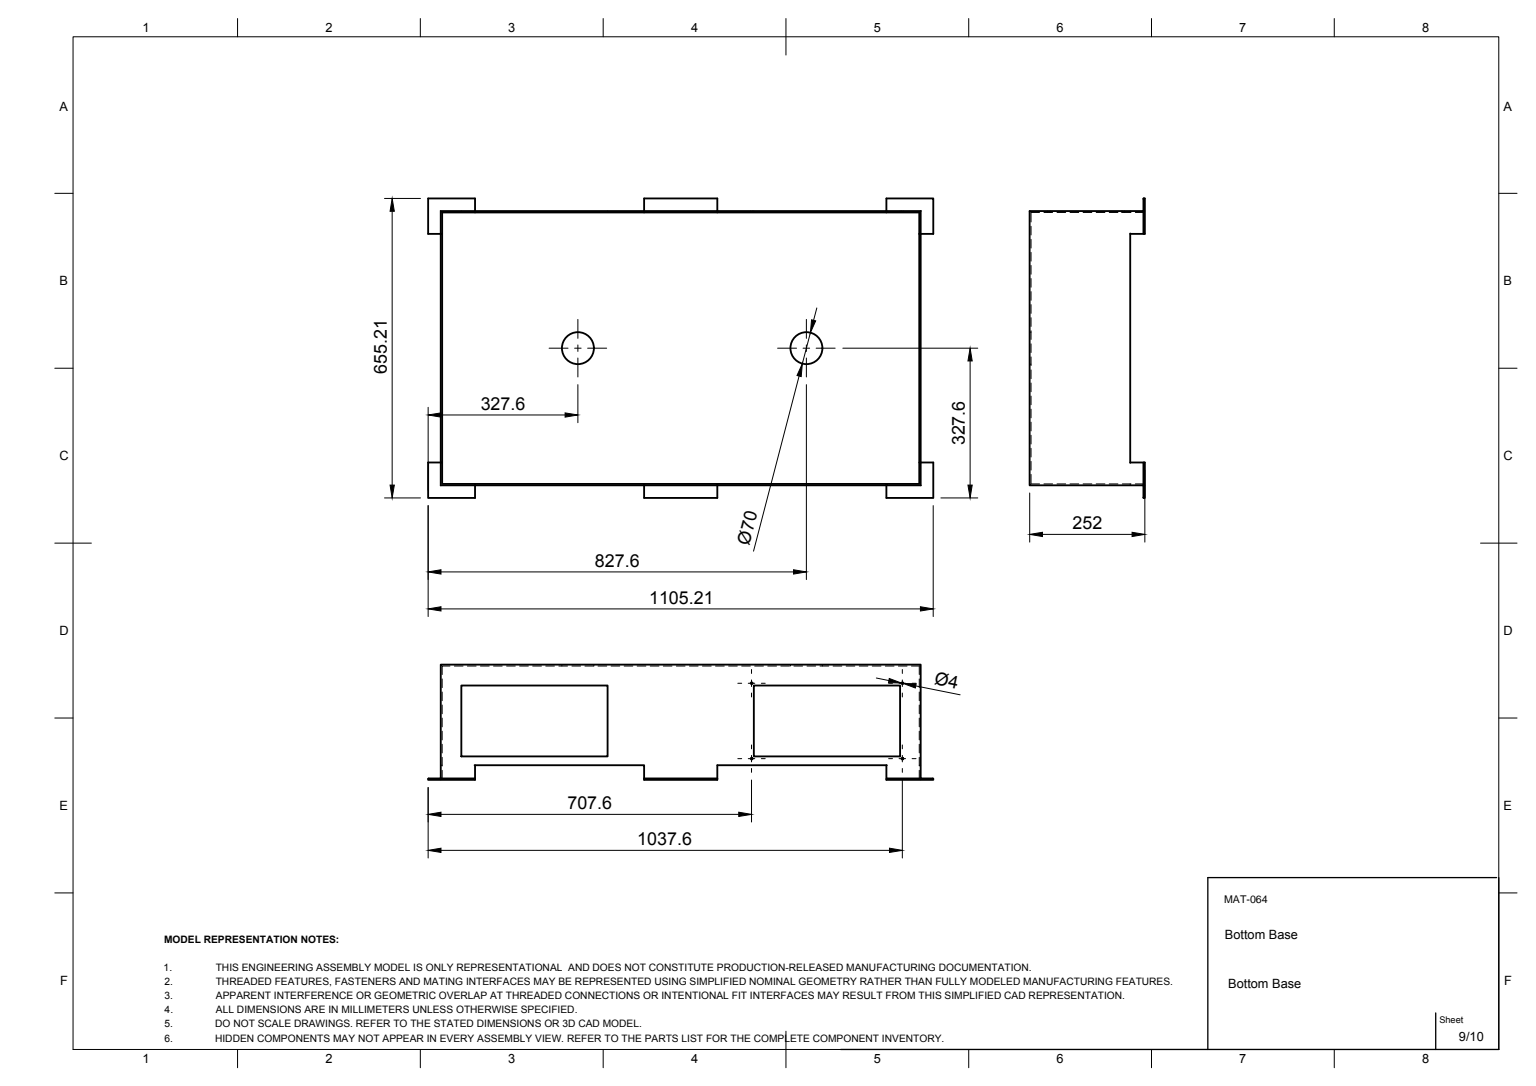
ISO-10303-21;
HEADER;
/* Generated by software containing ST-Developer
 * from STEP Tools, Inc. (www.steptools.com) 
 */

FILE_DESCRIPTION(
/* description */ (''),
/* implementation_level */ '2;1');

FILE_NAME(
/* name */ 
'Bottom Base.step',
/* time_stamp */ '2026-10-24T12:42:14-07:00',
/* author */ (''),
/* organization */ (''),
/* preprocessor_version */ 'ST-DEVELOPER v20.2',
/* originating_system */ 'Autodesk Translation Framework v15.15.0.0',
/* authorisation */ '');

FILE_SCHEMA (('AUTOMOTIVE_DESIGN { 1 0 10303 214 3 1 1 }'));
ENDSEC;

DATA;
#10=MECHANICAL_DESIGN_GEOMETRIC_PRESENTATION_REPRESENTATION('',(#66),#6789);
#54=SHAPE_REPRESENTATION_RELATIONSHIP('SRR','None',#6821,#60);
#60=ADVANCED_BREP_SHAPE_REPRESENTATION('',(#72),#6783);
#66=STYLED_ITEM('',(#6863),#72);
#72=MANIFOLD_SOLID_BREP('Bottom Base',#3961);
#78=TOROIDAL_SURFACE('',#4150,2.,1.);
#79=TOROIDAL_SURFACE('',#4160,2.,1.);
#80=TOROIDAL_SURFACE('',#4170,2.,1.);
#81=TOROIDAL_SURFACE('',#4180,2.,1.);
#82=TOROIDAL_SURFACE('',#4190,2.,1.);
#83=TOROIDAL_SURFACE('',#4200,2.,1.);
#84=TOROIDAL_SURFACE('',#4208,2.,1.);
#85=TOROIDAL_SURFACE('',#4220,2.,1.);
#92=ELLIPSE('',#4145,1.41421356237309,1.);
#93=ELLIPSE('',#4149,1.41421356237309,1.);
#94=ELLIPSE('',#4153,1.41421356237309,1.);
#95=ELLIPSE('',#4155,1.41421356237309,1.);
#96=ELLIPSE('',#4165,1.4142135623731,1.);
#97=ELLIPSE('',#4169,1.41421356237309,1.);
#98=ELLIPSE('',#4173,1.41421356237309,1.);
#99=ELLIPSE('',#4175,1.41421356237309,1.);
#100=ELLIPSE('',#4185,1.41421356237309,1.);
#101=ELLIPSE('',#4189,1.41421356237309,1.);
#102=ELLIPSE('',#4193,1.41421356237309,1.);
#103=ELLIPSE('',#4195,1.41421356237309,1.);
#104=ELLIPSE('',#4206,1.41421356237309,1.);
#105=ELLIPSE('',#4211,1.41421356237309,1.);
#106=ELLIPSE('',#4213,1.4142135623731,1.);
#107=ELLIPSE('',#4215,1.4142135623731,1.);
#108=CYLINDRICAL_SURFACE('',#4093,2.);
#109=CYLINDRICAL_SURFACE('',#4094,2.);
#110=CYLINDRICAL_SURFACE('',#4095,2.);
#111=CYLINDRICAL_SURFACE('',#4096,2.);
#112=CYLINDRICAL_SURFACE('',#4143,1.);
#113=CYLINDRICAL_SURFACE('',#4146,1.);
#114=CYLINDRICAL_SURFACE('',#4148,1.);
#115=CYLINDRICAL_SURFACE('',#4152,1.);
#116=CYLINDRICAL_SURFACE('',#4154,1.);
#117=CYLINDRICAL_SURFACE('',#4156,1.);
#118=CYLINDRICAL_SURFACE('',#4158,1.);
#119=CYLINDRICAL_SURFACE('',#4162,1.);
#120=CYLINDRICAL_SURFACE('',#4163,1.);
#121=CYLINDRICAL_SURFACE('',#4166,1.);
#122=CYLINDRICAL_SURFACE('',#4168,1.);
#123=CYLINDRICAL_SURFACE('',#4172,1.);
#124=CYLINDRICAL_SURFACE('',#4174,1.);
#125=CYLINDRICAL_SURFACE('',#4176,1.);
#126=CYLINDRICAL_SURFACE('',#4178,1.);
#127=CYLINDRICAL_SURFACE('',#4182,1.);
#128=CYLINDRICAL_SURFACE('',#4183,1.);
#129=CYLINDRICAL_SURFACE('',#4186,1.);
#130=CYLINDRICAL_SURFACE('',#4188,1.);
#131=CYLINDRICAL_SURFACE('',#4192,1.);
#132=CYLINDRICAL_SURFACE('',#4194,1.);
#133=CYLINDRICAL_SURFACE('',#4196,1.);
#134=CYLINDRICAL_SURFACE('',#4198,1.);
#135=CYLINDRICAL_SURFACE('',#4202,1.);
#136=CYLINDRICAL_SURFACE('',#4203,1.);
#137=CYLINDRICAL_SURFACE('',#4205,1.);
#138=CYLINDRICAL_SURFACE('',#4210,1.);
#139=CYLINDRICAL_SURFACE('',#4212,1.);
#140=CYLINDRICAL_SURFACE('',#4214,1.);
#141=CYLINDRICAL_SURFACE('',#4216,1.);
#142=CYLINDRICAL_SURFACE('',#4218,1.);
#143=CYLINDRICAL_SURFACE('',#4222,1.);
#144=CYLINDRICAL_SURFACE('',#4223,35.);
#145=CYLINDRICAL_SURFACE('',#4224,35.);
#185=FACE_BOUND('',#612,.T.);
#186=FACE_BOUND('',#613,.T.);
#187=FACE_BOUND('',#614,.T.);
#188=FACE_BOUND('',#615,.T.);
#189=FACE_BOUND('',#616,.T.);
#190=FACE_BOUND('',#617,.T.);
#191=FACE_BOUND('',#624,.T.);
#192=FACE_BOUND('',#625,.T.);
#193=FACE_BOUND('',#626,.T.);
#194=FACE_BOUND('',#627,.T.);
#195=FACE_BOUND('',#628,.T.);
#196=FACE_BOUND('',#629,.T.);
#197=FACE_BOUND('',#635,.T.);
#198=FACE_BOUND('',#636,.T.);
#199=FACE_BOUND('',#641,.T.);
#200=FACE_BOUND('',#642,.T.);
#242=CIRCLE('',#4038,2.);
#243=CIRCLE('',#4039,2.);
#244=CIRCLE('',#4040,2.);
#245=CIRCLE('',#4041,2.);
#246=CIRCLE('',#4048,2.);
#247=CIRCLE('',#4049,2.);
#248=CIRCLE('',#4050,2.);
#249=CIRCLE('',#4051,2.);
#250=CIRCLE('',#4057,35.);
#251=CIRCLE('',#4058,35.);
#252=CIRCLE('',#4063,35.);
#253=CIRCLE('',#4064,35.);
#254=CIRCLE('',#4067,1.);
#255=CIRCLE('',#4069,2.);
#256=CIRCLE('',#4071,2.);
#257=CIRCLE('',#4073,1.);
#258=CIRCLE('',#4077,1.);
#259=CIRCLE('',#4079,2.);
#260=CIRCLE('',#4082,2.);
#261=CIRCLE('',#4084,1.);
#262=CIRCLE('',#4098,2.);
#263=CIRCLE('',#4100,1.);
#264=CIRCLE('',#4101,1.);
#265=CIRCLE('',#4103,2.);
#266=CIRCLE('',#4105,2.);
#267=CIRCLE('',#4107,1.);
#268=CIRCLE('',#4108,1.);
#269=CIRCLE('',#4110,2.);
#270=CIRCLE('',#4144,1.);
#271=CIRCLE('',#4147,1.);
#272=CIRCLE('',#4151,1.);
#273=CIRCLE('',#4157,1.);
#274=CIRCLE('',#4159,1.);
#275=CIRCLE('',#4161,1.);
#276=CIRCLE('',#4164,1.);
#277=CIRCLE('',#4167,1.);
#278=CIRCLE('',#4171,1.);
#279=CIRCLE('',#4177,1.);
#280=CIRCLE('',#4179,1.);
#281=CIRCLE('',#4181,1.);
#282=CIRCLE('',#4184,1.);
#283=CIRCLE('',#4187,1.);
#284=CIRCLE('',#4191,1.);
#285=CIRCLE('',#4197,1.);
#286=CIRCLE('',#4199,1.);
#287=CIRCLE('',#4201,1.);
#288=CIRCLE('',#4204,1.);
#289=CIRCLE('',#4207,1.);
#290=CIRCLE('',#4209,1.);
#291=CIRCLE('',#4217,1.);
#292=CIRCLE('',#4219,1.);
#293=CIRCLE('',#4221,1.);
#394=FACE_OUTER_BOUND('',#611,.T.);
#395=FACE_OUTER_BOUND('',#618,.T.);
#396=FACE_OUTER_BOUND('',#619,.T.);
#397=FACE_OUTER_BOUND('',#620,.T.);
#398=FACE_OUTER_BOUND('',#621,.T.);
#399=FACE_OUTER_BOUND('',#622,.T.);
#400=FACE_OUTER_BOUND('',#623,.T.);
#401=FACE_OUTER_BOUND('',#630,.T.);
#402=FACE_OUTER_BOUND('',#631,.T.);
#403=FACE_OUTER_BOUND('',#632,.T.);
#404=FACE_OUTER_BOUND('',#633,.T.);
#405=FACE_OUTER_BOUND('',#634,.T.);
#406=FACE_OUTER_BOUND('',#637,.T.);
#407=FACE_OUTER_BOUND('',#638,.T.);
#408=FACE_OUTER_BOUND('',#639,.T.);
#409=FACE_OUTER_BOUND('',#640,.T.);
#410=FACE_OUTER_BOUND('',#643,.T.);
#411=FACE_OUTER_BOUND('',#644,.T.);
#412=FACE_OUTER_BOUND('',#645,.T.);
#413=FACE_OUTER_BOUND('',#646,.T.);
#414=FACE_OUTER_BOUND('',#647,.T.);
#415=FACE_OUTER_BOUND('',#648,.T.);
#416=FACE_OUTER_BOUND('',#649,.T.);
#417=FACE_OUTER_BOUND('',#650,.T.);
#418=FACE_OUTER_BOUND('',#651,.T.);
#419=FACE_OUTER_BOUND('',#652,.T.);
#420=FACE_OUTER_BOUND('',#653,.T.);
#421=FACE_OUTER_BOUND('',#654,.T.);
#422=FACE_OUTER_BOUND('',#655,.T.);
#423=FACE_OUTER_BOUND('',#656,.T.);
#424=FACE_OUTER_BOUND('',#657,.T.);
#425=FACE_OUTER_BOUND('',#658,.T.);
#426=FACE_OUTER_BOUND('',#659,.T.);
#427=FACE_OUTER_BOUND('',#660,.T.);
#428=FACE_OUTER_BOUND('',#661,.T.);
#429=FACE_OUTER_BOUND('',#662,.T.);
#430=FACE_OUTER_BOUND('',#663,.T.);
#431=FACE_OUTER_BOUND('',#664,.T.);
#432=FACE_OUTER_BOUND('',#665,.T.);
#433=FACE_OUTER_BOUND('',#666,.T.);
#434=FACE_OUTER_BOUND('',#667,.T.);
#435=FACE_OUTER_BOUND('',#668,.T.);
#436=FACE_OUTER_BOUND('',#669,.T.);
#437=FACE_OUTER_BOUND('',#670,.T.);
#438=FACE_OUTER_BOUND('',#671,.T.);
#439=FACE_OUTER_BOUND('',#672,.T.);
#440=FACE_OUTER_BOUND('',#673,.T.);
#441=FACE_OUTER_BOUND('',#674,.T.);
#442=FACE_OUTER_BOUND('',#675,.T.);
#443=FACE_OUTER_BOUND('',#676,.T.);
#444=FACE_OUTER_BOUND('',#677,.T.);
#445=FACE_OUTER_BOUND('',#678,.T.);
#446=FACE_OUTER_BOUND('',#679,.T.);
#447=FACE_OUTER_BOUND('',#680,.T.);
#448=FACE_OUTER_BOUND('',#681,.T.);
#449=FACE_OUTER_BOUND('',#682,.T.);
#450=FACE_OUTER_BOUND('',#683,.T.);
#451=FACE_OUTER_BOUND('',#684,.T.);
#452=FACE_OUTER_BOUND('',#685,.T.);
#453=FACE_OUTER_BOUND('',#686,.T.);
#454=FACE_OUTER_BOUND('',#687,.T.);
#455=FACE_OUTER_BOUND('',#688,.T.);
#456=FACE_OUTER_BOUND('',#689,.T.);
#457=FACE_OUTER_BOUND('',#690,.T.);
#458=FACE_OUTER_BOUND('',#691,.T.);
#459=FACE_OUTER_BOUND('',#692,.T.);
#460=FACE_OUTER_BOUND('',#693,.T.);
#461=FACE_OUTER_BOUND('',#694,.T.);
#462=FACE_OUTER_BOUND('',#695,.T.);
#463=FACE_OUTER_BOUND('',#696,.T.);
#464=FACE_OUTER_BOUND('',#697,.T.);
#465=FACE_OUTER_BOUND('',#698,.T.);
#466=FACE_OUTER_BOUND('',#699,.T.);
#467=FACE_OUTER_BOUND('',#700,.T.);
#468=FACE_OUTER_BOUND('',#701,.T.);
#469=FACE_OUTER_BOUND('',#702,.T.);
#470=FACE_OUTER_BOUND('',#703,.T.);
#471=FACE_OUTER_BOUND('',#704,.T.);
#472=FACE_OUTER_BOUND('',#705,.T.);
#473=FACE_OUTER_BOUND('',#706,.T.);
#474=FACE_OUTER_BOUND('',#707,.T.);
#475=FACE_OUTER_BOUND('',#708,.T.);
#476=FACE_OUTER_BOUND('',#709,.T.);
#477=FACE_OUTER_BOUND('',#710,.T.);
#478=FACE_OUTER_BOUND('',#711,.T.);
#479=FACE_OUTER_BOUND('',#712,.T.);
#480=FACE_OUTER_BOUND('',#713,.T.);
#481=FACE_OUTER_BOUND('',#714,.T.);
#482=FACE_OUTER_BOUND('',#715,.T.);
#483=FACE_OUTER_BOUND('',#716,.T.);
#484=FACE_OUTER_BOUND('',#717,.T.);
#485=FACE_OUTER_BOUND('',#718,.T.);
#486=FACE_OUTER_BOUND('',#719,.T.);
#487=FACE_OUTER_BOUND('',#720,.T.);
#488=FACE_OUTER_BOUND('',#721,.T.);
#489=FACE_OUTER_BOUND('',#722,.T.);
#490=FACE_OUTER_BOUND('',#723,.T.);
#491=FACE_OUTER_BOUND('',#724,.T.);
#492=FACE_OUTER_BOUND('',#725,.T.);
#493=FACE_OUTER_BOUND('',#726,.T.);
#494=FACE_OUTER_BOUND('',#727,.T.);
#495=FACE_OUTER_BOUND('',#728,.T.);
#496=FACE_OUTER_BOUND('',#729,.T.);
#497=FACE_OUTER_BOUND('',#730,.T.);
#498=FACE_OUTER_BOUND('',#731,.T.);
#499=FACE_OUTER_BOUND('',#732,.T.);
#500=FACE_OUTER_BOUND('',#733,.T.);
#501=FACE_OUTER_BOUND('',#734,.T.);
#502=FACE_OUTER_BOUND('',#735,.T.);
#503=FACE_OUTER_BOUND('',#736,.T.);
#504=FACE_OUTER_BOUND('',#737,.T.);
#505=FACE_OUTER_BOUND('',#738,.T.);
#506=FACE_OUTER_BOUND('',#739,.T.);
#507=FACE_OUTER_BOUND('',#740,.T.);
#508=FACE_OUTER_BOUND('',#741,.T.);
#509=FACE_OUTER_BOUND('',#742,.T.);
#510=FACE_OUTER_BOUND('',#743,.T.);
#511=FACE_OUTER_BOUND('',#744,.T.);
#512=FACE_OUTER_BOUND('',#745,.T.);
#513=FACE_OUTER_BOUND('',#746,.T.);
#611=EDGE_LOOP('',(#2533,#2534,#2535,#2536,#2537,#2538,#2539,#2540,#2541,
#2542,#2543,#2544));
#612=EDGE_LOOP('',(#2545));
#613=EDGE_LOOP('',(#2546));
#614=EDGE_LOOP('',(#2547));
#615=EDGE_LOOP('',(#2548));
#616=EDGE_LOOP('',(#2549,#2550,#2551,#2552));
#617=EDGE_LOOP('',(#2553,#2554,#2555,#2556));
#618=EDGE_LOOP('',(#2557,#2558,#2559,#2560,#2561,#2562,#2563,#2564));
#619=EDGE_LOOP('',(#2565,#2566,#2567,#2568,#2569,#2570,#2571,#2572,#2573,
#2574,#2575,#2576));
#620=EDGE_LOOP('',(#2577,#2578,#2579,#2580,#2581,#2582,#2583,#2584));
#621=EDGE_LOOP('',(#2585,#2586,#2587,#2588,#2589,#2590));
#622=EDGE_LOOP('',(#2591,#2592,#2593,#2594,#2595,#2596));
#623=EDGE_LOOP('',(#2597,#2598,#2599,#2600,#2601,#2602,#2603,#2604,#2605,
#2606,#2607,#2608));
#624=EDGE_LOOP('',(#2609,#2610,#2611,#2612));
#625=EDGE_LOOP('',(#2613));
#626=EDGE_LOOP('',(#2614));
#627=EDGE_LOOP('',(#2615));
#628=EDGE_LOOP('',(#2616));
#629=EDGE_LOOP('',(#2617,#2618,#2619,#2620));
#630=EDGE_LOOP('',(#2621,#2622,#2623,#2624));
#631=EDGE_LOOP('',(#2625,#2626,#2627,#2628));
#632=EDGE_LOOP('',(#2629,#2630,#2631,#2632,#2633,#2634));
#633=EDGE_LOOP('',(#2635,#2636,#2637,#2638,#2639,#2640));
#634=EDGE_LOOP('',(#2641,#2642,#2643,#2644));
#635=EDGE_LOOP('',(#2645));
#636=EDGE_LOOP('',(#2646));
#637=EDGE_LOOP('',(#2647,#2648,#2649,#2650,#2651,#2652,#2653,#2654));
#638=EDGE_LOOP('',(#2655,#2656,#2657,#2658,#2659,#2660,#2661,#2662,#2663,
#2664,#2665,#2666));
#639=EDGE_LOOP('',(#2667,#2668,#2669,#2670,#2671,#2672,#2673,#2674));
#640=EDGE_LOOP('',(#2675,#2676,#2677,#2678));
#641=EDGE_LOOP('',(#2679));
#642=EDGE_LOOP('',(#2680));
#643=EDGE_LOOP('',(#2681,#2682,#2683,#2684,#2685,#2686,#2687,#2688));
#644=EDGE_LOOP('',(#2689,#2690,#2691,#2692,#2693));
#645=EDGE_LOOP('',(#2694,#2695,#2696,#2697,#2698,#2699,#2700,#2701,#2702));
#646=EDGE_LOOP('',(#2703,#2704,#2705,#2706,#2707,#2708,#2709,#2710,#2711));
#647=EDGE_LOOP('',(#2712,#2713,#2714,#2715,#2716));
#648=EDGE_LOOP('',(#2717,#2718,#2719,#2720,#2721,#2722,#2723,#2724));
#649=EDGE_LOOP('',(#2725,#2726,#2727,#2728,#2729,#2730,#2731,#2732));
#650=EDGE_LOOP('',(#2733,#2734,#2735,#2736,#2737));
#651=EDGE_LOOP('',(#2738,#2739,#2740,#2741,#2742,#2743,#2744,#2745,#2746));
#652=EDGE_LOOP('',(#2747,#2748,#2749,#2750,#2751,#2752,#2753,#2754));
#653=EDGE_LOOP('',(#2755,#2756,#2757,#2758,#2759,#2760,#2761,#2762,#2763));
#654=EDGE_LOOP('',(#2764,#2765,#2766,#2767,#2768));
#655=EDGE_LOOP('',(#2769,#2770,#2771,#2772));
#656=EDGE_LOOP('',(#2773,#2774,#2775,#2776));
#657=EDGE_LOOP('',(#2777,#2778,#2779,#2780));
#658=EDGE_LOOP('',(#2781,#2782,#2783,#2784));
#659=EDGE_LOOP('',(#2785,#2786,#2787,#2788));
#660=EDGE_LOOP('',(#2789,#2790,#2791,#2792));
#661=EDGE_LOOP('',(#2793,#2794,#2795,#2796));
#662=EDGE_LOOP('',(#2797,#2798,#2799,#2800));
#663=EDGE_LOOP('',(#2801,#2802,#2803,#2804));
#664=EDGE_LOOP('',(#2805,#2806,#2807,#2808));
#665=EDGE_LOOP('',(#2809,#2810,#2811,#2812));
#666=EDGE_LOOP('',(#2813,#2814,#2815,#2816));
#667=EDGE_LOOP('',(#2817,#2818,#2819,#2820,#2821,#2822,#2823,#2824,#2825));
#668=EDGE_LOOP('',(#2826,#2827,#2828,#2829,#2830,#2831));
#669=EDGE_LOOP('',(#2832,#2833,#2834,#2835,#2836,#2837,#2838,#2839,#2840));
#670=EDGE_LOOP('',(#2841,#2842,#2843,#2844,#2845,#2846,#2847,#2848,#2849));
#671=EDGE_LOOP('',(#2850,#2851,#2852,#2853,#2854,#2855));
#672=EDGE_LOOP('',(#2856,#2857,#2858,#2859,#2860,#2861,#2862,#2863,#2864));
#673=EDGE_LOOP('',(#2865,#2866,#2867,#2868));
#674=EDGE_LOOP('',(#2869,#2870,#2871,#2872));
#675=EDGE_LOOP('',(#2873,#2874,#2875,#2876));
#676=EDGE_LOOP('',(#2877,#2878,#2879,#2880));
#677=EDGE_LOOP('',(#2881,#2882,#2883,#2884,#2885,#2886));
#678=EDGE_LOOP('',(#2887,#2888,#2889,#2890,#2891,#2892));
#679=EDGE_LOOP('',(#2893,#2894,#2895,#2896));
#680=EDGE_LOOP('',(#2897,#2898,#2899,#2900));
#681=EDGE_LOOP('',(#2901,#2902,#2903,#2904));
#682=EDGE_LOOP('',(#2905,#2906,#2907,#2908));
#683=EDGE_LOOP('',(#2909,#2910,#2911,#2912,#2913,#2914));
#684=EDGE_LOOP('',(#2915,#2916,#2917,#2918,#2919,#2920));
#685=EDGE_LOOP('',(#2921,#2922,#2923,#2924));
#686=EDGE_LOOP('',(#2925,#2926,#2927,#2928));
#687=EDGE_LOOP('',(#2929,#2930,#2931,#2932));
#688=EDGE_LOOP('',(#2933,#2934,#2935,#2936));
#689=EDGE_LOOP('',(#2937,#2938,#2939,#2940,#2941,#2942));
#690=EDGE_LOOP('',(#2943,#2944,#2945,#2946,#2947,#2948));
#691=EDGE_LOOP('',(#2949,#2950,#2951,#2952));
#692=EDGE_LOOP('',(#2953,#2954,#2955,#2956));
#693=EDGE_LOOP('',(#2957,#2958,#2959,#2960));
#694=EDGE_LOOP('',(#2961,#2962,#2963,#2964));
#695=EDGE_LOOP('',(#2965,#2966,#2967,#2968,#2969,#2970));
#696=EDGE_LOOP('',(#2971,#2972,#2973,#2974,#2975,#2976));
#697=EDGE_LOOP('',(#2977,#2978,#2979,#2980));
#698=EDGE_LOOP('',(#2981,#2982,#2983,#2984));
#699=EDGE_LOOP('',(#2985,#2986,#2987,#2988));
#700=EDGE_LOOP('',(#2989,#2990,#2991,#2992));
#701=EDGE_LOOP('',(#2993,#2994,#2995,#2996));
#702=EDGE_LOOP('',(#2997,#2998,#2999,#3000));
#703=EDGE_LOOP('',(#3001,#3002,#3003,#3004));
#704=EDGE_LOOP('',(#3005,#3006,#3007,#3008));
#705=EDGE_LOOP('',(#3009,#3010,#3011,#3012));
#706=EDGE_LOOP('',(#3013,#3014,#3015,#3016));
#707=EDGE_LOOP('',(#3017,#3018,#3019,#3020));
#708=EDGE_LOOP('',(#3021,#3022,#3023,#3024));
#709=EDGE_LOOP('',(#3025,#3026,#3027,#3028));
#710=EDGE_LOOP('',(#3029,#3030,#3031,#3032));
#711=EDGE_LOOP('',(#3033,#3034,#3035,#3036));
#712=EDGE_LOOP('',(#3037,#3038,#3039,#3040));
#713=EDGE_LOOP('',(#3041,#3042,#3043,#3044));
#714=EDGE_LOOP('',(#3045,#3046,#3047,#3048));
#715=EDGE_LOOP('',(#3049,#3050,#3051,#3052));
#716=EDGE_LOOP('',(#3053,#3054,#3055,#3056));
#717=EDGE_LOOP('',(#3057,#3058,#3059,#3060));
#718=EDGE_LOOP('',(#3061,#3062,#3063,#3064));
#719=EDGE_LOOP('',(#3065,#3066,#3067,#3068));
#720=EDGE_LOOP('',(#3069,#3070,#3071,#3072));
#721=EDGE_LOOP('',(#3073,#3074,#3075,#3076));
#722=EDGE_LOOP('',(#3077,#3078,#3079,#3080));
#723=EDGE_LOOP('',(#3081,#3082,#3083,#3084));
#724=EDGE_LOOP('',(#3085,#3086,#3087,#3088));
#725=EDGE_LOOP('',(#3089,#3090,#3091,#3092));
#726=EDGE_LOOP('',(#3093,#3094,#3095,#3096));
#727=EDGE_LOOP('',(#3097,#3098,#3099,#3100));
#728=EDGE_LOOP('',(#3101,#3102,#3103,#3104));
#729=EDGE_LOOP('',(#3105,#3106,#3107,#3108));
#730=EDGE_LOOP('',(#3109,#3110,#3111,#3112));
#731=EDGE_LOOP('',(#3113,#3114,#3115,#3116));
#732=EDGE_LOOP('',(#3117,#3118,#3119,#3120));
#733=EDGE_LOOP('',(#3121,#3122,#3123,#3124));
#734=EDGE_LOOP('',(#3125,#3126,#3127,#3128));
#735=EDGE_LOOP('',(#3129,#3130,#3131,#3132));
#736=EDGE_LOOP('',(#3133,#3134,#3135,#3136));
#737=EDGE_LOOP('',(#3137,#3138,#3139,#3140));
#738=EDGE_LOOP('',(#3141,#3142,#3143,#3144));
#739=EDGE_LOOP('',(#3145,#3146,#3147,#3148));
#740=EDGE_LOOP('',(#3149,#3150,#3151,#3152));
#741=EDGE_LOOP('',(#3153,#3154,#3155,#3156));
#742=EDGE_LOOP('',(#3157,#3158,#3159,#3160));
#743=EDGE_LOOP('',(#3161,#3162,#3163,#3164));
#744=EDGE_LOOP('',(#3165,#3166,#3167,#3168));
#745=EDGE_LOOP('',(#3169,#3170,#3171,#3172));
#746=EDGE_LOOP('',(#3173,#3174,#3175,#3176));
#885=LINE('',#5612,#1263);
#886=LINE('',#5614,#1264);
#887=LINE('',#5616,#1265);
#888=LINE('',#5618,#1266);
#889=LINE('',#5620,#1267);
#890=LINE('',#5622,#1268);
#891=LINE('',#5624,#1269);
#892=LINE('',#5626,#1270);
#893=LINE('',#5628,#1271);
#894=LINE('',#5630,#1272);
#895=LINE('',#5632,#1273);
#896=LINE('',#5633,#1274);
#897=LINE('',#5644,#1275);
#898=LINE('',#5646,#1276);
#899=LINE('',#5648,#1277);
#900=LINE('',#5649,#1278);
#901=LINE('',#5652,#1279);
#902=LINE('',#5654,#1280);
#903=LINE('',#5656,#1281);
#904=LINE('',#5657,#1282);
#905=LINE('',#5661,#1283);
#906=LINE('',#5663,#1284);
#907=LINE('',#5665,#1285);
#908=LINE('',#5666,#1286);
#909=LINE('',#5668,#1287);
#910=LINE('',#5670,#1288);
#911=LINE('',#5671,#1289);
#912=LINE('',#5675,#1290);
#913=LINE('',#5677,#1291);
#914=LINE('',#5678,#1292);
#915=LINE('',#5680,#1293);
#916=LINE('',#5682,#1294);
#917=LINE('',#5684,#1295);
#918=LINE('',#5686,#1296);
#919=LINE('',#5688,#1297);
#920=LINE('',#5690,#1298);
#921=LINE('',#5692,#1299);
#922=LINE('',#5693,#1300);
#923=LINE('',#5697,#1301);
#924=LINE('',#5699,#1302);
#925=LINE('',#5700,#1303);
#926=LINE('',#5701,#1304);
#927=LINE('',#5703,#1305);
#928=LINE('',#5704,#1306);
#929=LINE('',#5708,#1307);
#930=LINE('',#5710,#1308);
#931=LINE('',#5712,#1309);
#932=LINE('',#5714,#1310);
#933=LINE('',#5716,#1311);
#934=LINE('',#5717,#1312);
#935=LINE('',#5721,#1313);
#936=LINE('',#5723,#1314);
#937=LINE('',#5725,#1315);
#938=LINE('',#5727,#1316);
#939=LINE('',#5729,#1317);
#940=LINE('',#5730,#1318);
#941=LINE('',#5734,#1319);
#942=LINE('',#5736,#1320);
#943=LINE('',#5738,#1321);
#944=LINE('',#5740,#1322);
#945=LINE('',#5742,#1323);
#946=LINE('',#5744,#1324);
#947=LINE('',#5746,#1325);
#948=LINE('',#5748,#1326);
#949=LINE('',#5750,#1327);
#950=LINE('',#5752,#1328);
#951=LINE('',#5754,#1329);
#952=LINE('',#5755,#1330);
#953=LINE('',#5758,#1331);
#954=LINE('',#5760,#1332);
#955=LINE('',#5762,#1333);
#956=LINE('',#5763,#1334);
#957=LINE('',#5774,#1335);
#958=LINE('',#5776,#1336);
#959=LINE('',#5778,#1337);
#960=LINE('',#5779,#1338);
#961=LINE('',#5783,#1339);
#962=LINE('',#5785,#1340);
#963=LINE('',#5787,#1341);
#964=LINE('',#5788,#1342);
#965=LINE('',#5791,#1343);
#966=LINE('',#5793,#1344);
#967=LINE('',#5794,#1345);
#968=LINE('',#5798,#1346);
#969=LINE('',#5799,#1347);
#970=LINE('',#5801,#1348);
#971=LINE('',#5803,#1349);
#972=LINE('',#5804,#1350);
#973=LINE('',#5808,#1351);
#974=LINE('',#5810,#1352);
#975=LINE('',#5812,#1353);
#976=LINE('',#5813,#1354);
#977=LINE('',#5814,#1355);
#978=LINE('',#5822,#1356);
#979=LINE('',#5824,#1357);
#980=LINE('',#5825,#1358);
#981=LINE('',#5827,#1359);
#982=LINE('',#5828,#1360);
#983=LINE('',#5831,#1361);
#984=LINE('',#5833,#1362);
#985=LINE('',#5834,#1363);
#986=LINE('',#5836,#1364);
#987=LINE('',#5837,#1365);
#988=LINE('',#5839,#1366);
#989=LINE('',#5841,#1367);
#990=LINE('',#5842,#1368);
#991=LINE('',#5845,#1369);
#992=LINE('',#5847,#1370);
#993=LINE('',#5848,#1371);
#994=LINE('',#5849,#1372);
#995=LINE('',#5857,#1373);
#996=LINE('',#5859,#1374);
#997=LINE('',#5861,#1375);
#998=LINE('',#5862,#1376);
#999=LINE('',#5863,#1377);
#1000=LINE('',#5867,#1378);
#1001=LINE('',#5870,#1379);
#1002=LINE('',#5874,#1380);
#1003=LINE('',#5876,#1381);
#1004=LINE('',#5878,#1382);
#1005=LINE('',#5879,#1383);
#1006=LINE('',#5885,#1384);
#1007=LINE('',#5886,#1385);
#1008=LINE('',#5888,#1386);
#1009=LINE('',#5890,#1387);
#1010=LINE('',#5892,#1388);
#1011=LINE('',#5893,#1389);
#1012=LINE('',#5895,#1390);
#1013=LINE('',#5899,#1391);
#1014=LINE('',#5901,#1392);
#1015=LINE('',#5903,#1393);
#1016=LINE('',#5904,#1394);
#1017=LINE('',#5906,#1395);
#1018=LINE('',#5908,#1396);
#1019=LINE('',#5910,#1397);
#1020=LINE('',#5912,#1398);
#1021=LINE('',#5913,#1399);
#1022=LINE('',#5916,#1400);
#1023=LINE('',#5922,#1401);
#1024=LINE('',#5924,#1402);
#1025=LINE('',#5926,#1403);
#1026=LINE('',#5928,#1404);
#1027=LINE('',#5929,#1405);
#1028=LINE('',#5932,#1406);
#1029=LINE('',#5934,#1407);
#1030=LINE('',#5936,#1408);
#1031=LINE('',#5937,#1409);
#1032=LINE('',#5938,#1410);
#1033=LINE('',#5941,#1411);
#1034=LINE('',#5943,#1412);
#1035=LINE('',#5947,#1413);
#1036=LINE('',#5949,#1414);
#1037=LINE('',#5951,#1415);
#1038=LINE('',#5952,#1416);
#1039=LINE('',#5956,#1417);
#1040=LINE('',#5957,#1418);
#1041=LINE('',#5959,#1419);
#1042=LINE('',#5961,#1420);
#1043=LINE('',#5964,#1421);
#1044=LINE('',#5965,#1422);
#1045=LINE('',#5967,#1423);
#1046=LINE('',#5969,#1424);
#1047=LINE('',#5972,#1425);
#1048=LINE('',#5974,#1426);
#1049=LINE('',#5976,#1427);
#1050=LINE('',#5978,#1428);
#1051=LINE('',#5981,#1429);
#1052=LINE('',#5983,#1430);
#1053=LINE('',#5987,#1431);
#1054=LINE('',#5989,#1432);
#1055=LINE('',#5991,#1433);
#1056=LINE('',#5992,#1434);
#1057=LINE('',#5995,#1435);
#1058=LINE('',#6002,#1436);
#1059=LINE('',#6004,#1437);
#1060=LINE('',#6006,#1438);
#1061=LINE('',#6008,#1439);
#1062=LINE('',#6009,#1440);
#1063=LINE('',#6012,#1441);
#1064=LINE('',#6014,#1442);
#1065=LINE('',#6018,#1443);
#1066=LINE('',#6020,#1444);
#1067=LINE('',#6022,#1445);
#1068=LINE('',#6023,#1446);
#1069=LINE('',#6026,#1447);
#1070=LINE('',#6033,#1448);
#1071=LINE('',#6035,#1449);
#1072=LINE('',#6037,#1450);
#1073=LINE('',#6039,#1451);
#1074=LINE('',#6040,#1452);
#1075=LINE('',#6043,#1453);
#1076=LINE('',#6045,#1454);
#1077=LINE('',#6046,#1455);
#1078=LINE('',#6049,#1456);
#1079=LINE('',#6050,#1457);
#1080=LINE('',#6052,#1458);
#1081=LINE('',#6054,#1459);
#1082=LINE('',#6055,#1460);
#1083=LINE('',#6059,#1461);
#1084=LINE('',#6061,#1462);
#1085=LINE('',#6063,#1463);
#1086=LINE('',#6065,#1464);
#1087=LINE('',#6067,#1465);
#1088=LINE('',#6068,#1466);
#1089=LINE('',#6072,#1467);
#1090=LINE('',#6073,#1468);
#1091=LINE('',#6077,#1469);
#1092=LINE('',#6078,#1470);
#1093=LINE('',#6079,#1471);
#1094=LINE('',#6081,#1472);
#1095=LINE('',#6082,#1473);
#1096=LINE('',#6084,#1474);
#1097=LINE('',#6088,#1475);
#1098=LINE('',#6090,#1476);
#1099=LINE('',#6092,#1477);
#1100=LINE('',#6094,#1478);
#1101=LINE('',#6096,#1479);
#1102=LINE('',#6097,#1480);
#1103=LINE('',#6101,#1481);
#1104=LINE('',#6102,#1482);
#1105=LINE('',#6106,#1483);
#1106=LINE('',#6107,#1484);
#1107=LINE('',#6108,#1485);
#1108=LINE('',#6110,#1486);
#1109=LINE('',#6111,#1487);
#1110=LINE('',#6113,#1488);
#1111=LINE('',#6117,#1489);
#1112=LINE('',#6119,#1490);
#1113=LINE('',#6121,#1491);
#1114=LINE('',#6123,#1492);
#1115=LINE('',#6125,#1493);
#1116=LINE('',#6126,#1494);
#1117=LINE('',#6130,#1495);
#1118=LINE('',#6131,#1496);
#1119=LINE('',#6135,#1497);
#1120=LINE('',#6136,#1498);
#1121=LINE('',#6137,#1499);
#1122=LINE('',#6139,#1500);
#1123=LINE('',#6140,#1501);
#1124=LINE('',#6142,#1502);
#1125=LINE('',#6146,#1503);
#1126=LINE('',#6148,#1504);
#1127=LINE('',#6150,#1505);
#1128=LINE('',#6152,#1506);
#1129=LINE('',#6154,#1507);
#1130=LINE('',#6155,#1508);
#1131=LINE('',#6158,#1509);
#1132=LINE('',#6160,#1510);
#1133=LINE('',#6161,#1511);
#1134=LINE('',#6165,#1512);
#1135=LINE('',#6166,#1513);
#1136=LINE('',#6168,#1514);
#1137=LINE('',#6252,#1515);
#1138=LINE('',#6254,#1516);
#1263=VECTOR('',#4440,371.);
#1264=VECTOR('',#4441,28.0000000000002);
#1265=VECTOR('',#4442,73.9999999999999);
#1266=VECTOR('',#4443,248.);
#1267=VECTOR('',#4444,1050.);
#1268=VECTOR('',#4445,248.);
#1269=VECTOR('',#4446,74.0000000000001);
#1270=VECTOR('',#4447,28.0000000000002);
#1271=VECTOR('',#4448,371.);
#1272=VECTOR('',#4449,29.0000000000002);
#1273=VECTOR('',#4450,160.);
#1274=VECTOR('',#4451,29.0000000000002);
#1275=VECTOR('',#4460,155.);
#1276=VECTOR('',#4461,320.);
#1277=VECTOR('',#4462,155.);
#1278=VECTOR('',#4463,320.);
#1279=VECTOR('',#4464,320.);
#1280=VECTOR('',#4465,155.);
#1281=VECTOR('',#4466,320.);
#1282=VECTOR('',#4467,155.);
#1283=VECTOR('',#4470,28.);
#1284=VECTOR('',#4471,502.);
#1285=VECTOR('',#4472,28.0000000000002);
#1286=VECTOR('',#4473,49.);
#1287=VECTOR('',#4474,600.);
#1288=VECTOR('',#4475,248.);
#1289=VECTOR('',#4476,48.9999999999998);
#1290=VECTOR('',#4479,371.);
#1291=VECTOR('',#4480,28.0000000000002);
#1292=VECTOR('',#4481,73.9999999999999);
#1293=VECTOR('',#4482,1050.);
#1294=VECTOR('',#4483,248.);
#1295=VECTOR('',#4484,73.9999999999999);
#1296=VECTOR('',#4485,28.0000000000002);
#1297=VECTOR('',#4486,371.);
#1298=VECTOR('',#4487,29.0000000000002);
#1299=VECTOR('',#4488,160.);
#1300=VECTOR('',#4489,29.0000000000002);
#1301=VECTOR('',#4492,502.);
#1302=VECTOR('',#4493,28.);
#1303=VECTOR('',#4494,49.0000000000001);
#1304=VECTOR('',#4495,600.);
#1305=VECTOR('',#4496,48.9999999999998);
#1306=VECTOR('',#4497,28.0000000000002);
#1307=VECTOR('',#4500,3.00000000000011);
#1308=VECTOR('',#4501,49.9999999999997);
#1309=VECTOR('',#4502,74.9999999999999);
#1310=VECTOR('',#4503,3.00000000000001);
#1311=VECTOR('',#4504,71.9999999999999);
#1312=VECTOR('',#4505,46.9999999999998);
#1313=VECTOR('',#4508,3.00000000000011);
#1314=VECTOR('',#4509,47.0000000000001);
#1315=VECTOR('',#4510,71.9999999999999);
#1316=VECTOR('',#4511,3.00000000000001);
#1317=VECTOR('',#4512,75.);
#1318=VECTOR('',#4513,50.0000000000001);
#1319=VECTOR('',#4516,370.);
#1320=VECTOR('',#4517,30.0000000000001);
#1321=VECTOR('',#4518,160.);
#1322=VECTOR('',#4519,30.0000000000001);
#1323=VECTOR('',#4520,370.);
#1324=VECTOR('',#4521,30.0000000000001);
#1325=VECTOR('',#4522,72.);
#1326=VECTOR('',#4523,247.);
#1327=VECTOR('',#4524,1044.);
#1328=VECTOR('',#4525,247.);
#1329=VECTOR('',#4526,71.9999999999999);
#1330=VECTOR('',#4527,30.0000000000001);
#1331=VECTOR('',#4528,155.);
#1332=VECTOR('',#4529,320.);
#1333=VECTOR('',#4530,155.);
#1334=VECTOR('',#4531,320.);
#1335=VECTOR('',#4540,320.);
#1336=VECTOR('',#4541,155.);
#1337=VECTOR('',#4542,320.);
#1338=VECTOR('',#4543,155.);
#1339=VECTOR('',#4546,3.00000000000001);
#1340=VECTOR('',#4547,160.);
#1341=VECTOR('',#4548,3.00000000000001);
#1342=VECTOR('',#4549,160.);
#1343=VECTOR('',#4552,3.00000000000001);
#1344=VECTOR('',#4553,160.);
#1345=VECTOR('',#4554,3.00000000000001);
#1346=VECTOR('',#4557,2.99999999999997);
#1347=VECTOR('',#4558,47.);
#1348=VECTOR('',#4559,3.00000000000001);
#1349=VECTOR('',#4560,75.);
#1350=VECTOR('',#4561,50.);
#1351=VECTOR('',#4564,3.00000000000001);
#1352=VECTOR('',#4565,49.9999999999998);
#1353=VECTOR('',#4566,75.);
#1354=VECTOR('',#4567,3.00000000000001);
#1355=VECTOR('',#4568,46.9999999999998);
#1356=VECTOR('',#4577,30.);
#1357=VECTOR('',#4578,247.);
#1358=VECTOR('',#4579,594.);
#1359=VECTOR('',#4580,30.0000000000001);
#1360=VECTOR('',#4581,500.);
#1361=VECTOR('',#4584,30.0000000000001);
#1362=VECTOR('',#4585,370.);
#1363=VECTOR('',#4586,30.0000000000001);
#1364=VECTOR('',#4587,247.);
#1365=VECTOR('',#4588,1044.);
#1366=VECTOR('',#4589,30.0000000000001);
#1367=VECTOR('',#4590,370.);
#1368=VECTOR('',#4591,30.0000000000001);
#1369=VECTOR('',#4594,30.);
#1370=VECTOR('',#4595,500.);
#1371=VECTOR('',#4596,30.0000000000001);
#1372=VECTOR('',#4597,594.);
#1373=VECTOR('',#4606,2.00000000000003);
#1374=VECTOR('',#4607,27.6040069435298);
#1375=VECTOR('',#4608,2.99999999999997);
#1376=VECTOR('',#4609,27.6040069435298);
#1377=VECTOR('',#4610,3.00000000000001);
#1378=VECTOR('',#4615,1.99999999999999);
#1379=VECTOR('',#4618,28.0000000000002);
#1380=VECTOR('',#4621,26.6040069435298);
#1381=VECTOR('',#4622,2.00000000000003);
#1382=VECTOR('',#4623,27.6040069435297);
#1383=VECTOR('',#4624,2.00000000000003);
#1384=VECTOR('',#4629,28.0000000000002);
#1385=VECTOR('',#4630,1.99999999999999);
#1386=VECTOR('',#4631,2.00000000000003);
#1387=VECTOR('',#4632,27.6040069435297);
#1388=VECTOR('',#4633,2.00000000000003);
#1389=VECTOR('',#4634,26.6040069435298);
#1390=VECTOR('',#4637,3.00000000000001);
#1391=VECTOR('',#4642,27.6040069435298);
#1392=VECTOR('',#4643,2.99999999999997);
#1393=VECTOR('',#4644,27.6040069435298);
#1394=VECTOR('',#4645,2.00000000000003);
#1395=VECTOR('',#4648,3.00000000000001);
#1396=VECTOR('',#4649,27.6040069435298);
#1397=VECTOR('',#4650,2.99999999999997);
#1398=VECTOR('',#4651,27.6040069435298);
#1399=VECTOR('',#4652,2.00000000000003);
#1400=VECTOR('',#4655,1.99999999999999);
#1401=VECTOR('',#4662,28.0000000000002);
#1402=VECTOR('',#4663,2.00000000000003);
#1403=VECTOR('',#4664,27.6040069435297);
#1404=VECTOR('',#4665,2.00000000000003);
#1405=VECTOR('',#4666,26.6040069435298);
#1406=VECTOR('',#4669,2.00000000000003);
#1407=VECTOR('',#4670,27.6040069435298);
#1408=VECTOR('',#4671,2.99999999999997);
#1409=VECTOR('',#4672,27.6040069435298);
#1410=VECTOR('',#4673,3.00000000000001);
#1411=VECTOR('',#4676,1.99999999999999);
#1412=VECTOR('',#4677,28.0000000000002);
#1413=VECTOR('',#4680,26.6040069435298);
#1414=VECTOR('',#4681,2.00000000000003);
#1415=VECTOR('',#4682,27.6040069435297);
#1416=VECTOR('',#4683,2.00000000000003);
#1417=VECTOR('',#4690,3.00000000000001);
#1418=VECTOR('',#4691,3.00000000000001);
#1419=VECTOR('',#4694,3.00000000000001);
#1420=VECTOR('',#4697,3.00000000000001);
#1421=VECTOR('',#4702,3.00000000000001);
#1422=VECTOR('',#4703,3.00000000000001);
#1423=VECTOR('',#4706,3.00000000000001);
#1424=VECTOR('',#4709,3.00000000000001);
#1425=VECTOR('',#4714,2.);
#1426=VECTOR('',#4717,2.);
#1427=VECTOR('',#4720,2.);
#1428=VECTOR('',#4723,2.);
#1429=VECTOR('',#4726,1.99999999999999);
#1430=VECTOR('',#4727,28.0000000000002);
#1431=VECTOR('',#4730,26.6040069435297);
#1432=VECTOR('',#4731,2.00000000000003);
#1433=VECTOR('',#4732,27.6040069435296);
#1434=VECTOR('',#4733,2.00000000000003);
#1435=VECTOR('',#4736,1.99999999999999);
#1436=VECTOR('',#4745,28.);
#1437=VECTOR('',#4746,2.00000000000003);
#1438=VECTOR('',#4747,27.6040069435296);
#1439=VECTOR('',#4748,2.00000000000003);
#1440=VECTOR('',#4749,26.6040069435297);
#1441=VECTOR('',#4752,2.00000000000003);
#1442=VECTOR('',#4753,28.);
#1443=VECTOR('',#4756,26.6040069435299);
#1444=VECTOR('',#4757,2.00000000000003);
#1445=VECTOR('',#4758,27.6040069435297);
#1446=VECTOR('',#4759,2.00000000000003);
#1447=VECTOR('',#4762,2.00000000000017);
#1448=VECTOR('',#4771,28.0000000000002);
#1449=VECTOR('',#4772,2.00000000000003);
#1450=VECTOR('',#4773,27.6040069435297);
#1451=VECTOR('',#4774,2.00000000000003);
#1452=VECTOR('',#4775,26.6040069435299);
#1453=VECTOR('',#4778,102.60400694353);
#1454=VECTOR('',#4779,2.00000000000003);
#1455=VECTOR('',#4780,102.60400694353);
#1456=VECTOR('',#4783,2.00000000000003);
#1457=VECTOR('',#4784,75.);
#1458=VECTOR('',#4787,50.);
#1459=VECTOR('',#4790,77.6040069435298);
#1460=VECTOR('',#4791,77.6040069435298);
#1461=VECTOR('',#4794,25.6040069435298);
#1462=VECTOR('',#4795,75.6040069435298);
#1463=VECTOR('',#4796,100.60400694353);
#1464=VECTOR('',#4797,25.6040069435297);
#1465=VECTOR('',#4798,75.);
#1466=VECTOR('',#4799,50.);
#1467=VECTOR('',#4804,2.00000000000003);
#1468=VECTOR('',#4805,75.);
#1469=VECTOR('',#4808,2.00000000000003);
#1470=VECTOR('',#4809,102.60400694353);
#1471=VECTOR('',#4810,102.60400694353);
#1472=VECTOR('',#4813,77.6040069435298);
#1473=VECTOR('',#4814,77.6040069435298);
#1474=VECTOR('',#4817,50.);
#1475=VECTOR('',#4820,25.6040069435299);
#1476=VECTOR('',#4821,49.9999999999999);
#1477=VECTOR('',#4822,74.9999999999999);
#1478=VECTOR('',#4823,25.6040069435297);
#1479=VECTOR('',#4824,100.60400694353);
#1480=VECTOR('',#4825,75.6040069435296);
#1481=VECTOR('',#4830,2.00000000000003);
#1482=VECTOR('',#4831,50.);
#1483=VECTOR('',#4834,2.00000000000003);
#1484=VECTOR('',#4835,77.6040069435298);
#1485=VECTOR('',#4836,77.6040069435298);
#1486=VECTOR('',#4839,102.60400694353);
#1487=VECTOR('',#4840,102.60400694353);
#1488=VECTOR('',#4843,75.0000000000001);
#1489=VECTOR('',#4846,25.6040069435297);
#1490=VECTOR('',#4847,74.9999999999999);
#1491=VECTOR('',#4848,50.);
#1492=VECTOR('',#4849,25.6040069435297);
#1493=VECTOR('',#4850,75.6040069435298);
#1494=VECTOR('',#4851,100.60400694353);
#1495=VECTOR('',#4856,2.00000000000003);
#1496=VECTOR('',#4857,75.0000000000001);
#1497=VECTOR('',#4860,2.00000000000003);
#1498=VECTOR('',#4861,102.60400694353);
#1499=VECTOR('',#4862,102.60400694353);
#1500=VECTOR('',#4865,77.6040069435298);
#1501=VECTOR('',#4866,77.6040069435298);
#1502=VECTOR('',#4869,50.);
#1503=VECTOR('',#4872,25.6040069435297);
#1504=VECTOR('',#4873,49.9999999999998);
#1505=VECTOR('',#4874,74.9999999999999);
#1506=VECTOR('',#4875,25.6040069435297);
#1507=VECTOR('',#4876,100.60400694353);
#1508=VECTOR('',#4877,75.6040069435296);
#1509=VECTOR('',#4882,160.);
#1510=VECTOR('',#4885,160.);
#1511=VECTOR('',#4886,160.);
#1512=VECTOR('',#4893,160.);
#1513=VECTOR('',#4894,160.);
#1514=VECTOR('',#4897,160.);
#1515=VECTOR('',#5064,35.);
#1516=VECTOR('',#5067,35.);
#1641=VERTEX_POINT('',#5610);
#1642=VERTEX_POINT('',#5611);
#1643=VERTEX_POINT('',#5613);
#1644=VERTEX_POINT('',#5615);
#1645=VERTEX_POINT('',#5617);
#1646=VERTEX_POINT('',#5619);
#1647=VERTEX_POINT('',#5621);
#1648=VERTEX_POINT('',#5623);
#1649=VERTEX_POINT('',#5625);
#1650=VERTEX_POINT('',#5627);
#1651=VERTEX_POINT('',#5629);
#1652=VERTEX_POINT('',#5631);
#1653=VERTEX_POINT('',#5634);
#1654=VERTEX_POINT('',#5636);
#1655=VERTEX_POINT('',#5638);
#1656=VERTEX_POINT('',#5640);
#1657=VERTEX_POINT('',#5642);
#1658=VERTEX_POINT('',#5643);
#1659=VERTEX_POINT('',#5645);
#1660=VERTEX_POINT('',#5647);
#1661=VERTEX_POINT('',#5650);
#1662=VERTEX_POINT('',#5651);
#1663=VERTEX_POINT('',#5653);
#1664=VERTEX_POINT('',#5655);
#1665=VERTEX_POINT('',#5659);
#1666=VERTEX_POINT('',#5660);
#1667=VERTEX_POINT('',#5662);
#1668=VERTEX_POINT('',#5664);
#1669=VERTEX_POINT('',#5667);
#1670=VERTEX_POINT('',#5669);
#1671=VERTEX_POINT('',#5673);
#1672=VERTEX_POINT('',#5674);
#1673=VERTEX_POINT('',#5676);
#1674=VERTEX_POINT('',#5679);
#1675=VERTEX_POINT('',#5681);
#1676=VERTEX_POINT('',#5683);
#1677=VERTEX_POINT('',#5685);
#1678=VERTEX_POINT('',#5687);
#1679=VERTEX_POINT('',#5689);
#1680=VERTEX_POINT('',#5691);
#1681=VERTEX_POINT('',#5695);
#1682=VERTEX_POINT('',#5696);
#1683=VERTEX_POINT('',#5698);
#1684=VERTEX_POINT('',#5702);
#1685=VERTEX_POINT('',#5706);
#1686=VERTEX_POINT('',#5707);
#1687=VERTEX_POINT('',#5709);
#1688=VERTEX_POINT('',#5711);
#1689=VERTEX_POINT('',#5713);
#1690=VERTEX_POINT('',#5715);
#1691=VERTEX_POINT('',#5719);
#1692=VERTEX_POINT('',#5720);
#1693=VERTEX_POINT('',#5722);
#1694=VERTEX_POINT('',#5724);
#1695=VERTEX_POINT('',#5726);
#1696=VERTEX_POINT('',#5728);
#1697=VERTEX_POINT('',#5732);
#1698=VERTEX_POINT('',#5733);
#1699=VERTEX_POINT('',#5735);
#1700=VERTEX_POINT('',#5737);
#1701=VERTEX_POINT('',#5739);
#1702=VERTEX_POINT('',#5741);
#1703=VERTEX_POINT('',#5743);
#1704=VERTEX_POINT('',#5745);
#1705=VERTEX_POINT('',#5747);
#1706=VERTEX_POINT('',#5749);
#1707=VERTEX_POINT('',#5751);
#1708=VERTEX_POINT('',#5753);
#1709=VERTEX_POINT('',#5756);
#1710=VERTEX_POINT('',#5757);
#1711=VERTEX_POINT('',#5759);
#1712=VERTEX_POINT('',#5761);
#1713=VERTEX_POINT('',#5764);
#1714=VERTEX_POINT('',#5766);
#1715=VERTEX_POINT('',#5768);
#1716=VERTEX_POINT('',#5770);
#1717=VERTEX_POINT('',#5772);
#1718=VERTEX_POINT('',#5773);
#1719=VERTEX_POINT('',#5775);
#1720=VERTEX_POINT('',#5777);
#1721=VERTEX_POINT('',#5781);
#1722=VERTEX_POINT('',#5782);
#1723=VERTEX_POINT('',#5784);
#1724=VERTEX_POINT('',#5786);
#1725=VERTEX_POINT('',#5790);
#1726=VERTEX_POINT('',#5792);
#1727=VERTEX_POINT('',#5796);
#1728=VERTEX_POINT('',#5797);
#1729=VERTEX_POINT('',#5800);
#1730=VERTEX_POINT('',#5802);
#1731=VERTEX_POINT('',#5806);
#1732=VERTEX_POINT('',#5807);
#1733=VERTEX_POINT('',#5809);
#1734=VERTEX_POINT('',#5811);
#1735=VERTEX_POINT('',#5816);
#1736=VERTEX_POINT('',#5818);
#1737=VERTEX_POINT('',#5821);
#1738=VERTEX_POINT('',#5823);
#1739=VERTEX_POINT('',#5826);
#1740=VERTEX_POINT('',#5830);
#1741=VERTEX_POINT('',#5832);
#1742=VERTEX_POINT('',#5835);
#1743=VERTEX_POINT('',#5838);
#1744=VERTEX_POINT('',#5840);
#1745=VERTEX_POINT('',#5844);
#1746=VERTEX_POINT('',#5846);
#1747=VERTEX_POINT('',#5851);
#1748=VERTEX_POINT('',#5853);
#1749=VERTEX_POINT('',#5856);
#1750=VERTEX_POINT('',#5858);
#1751=VERTEX_POINT('',#5860);
#1752=VERTEX_POINT('',#5865);
#1753=VERTEX_POINT('',#5869);
#1754=VERTEX_POINT('',#5871);
#1755=VERTEX_POINT('',#5873);
#1756=VERTEX_POINT('',#5875);
#1757=VERTEX_POINT('',#5877);
#1758=VERTEX_POINT('',#5881);
#1759=VERTEX_POINT('',#5882);
#1760=VERTEX_POINT('',#5884);
#1761=VERTEX_POINT('',#5887);
#1762=VERTEX_POINT('',#5889);
#1763=VERTEX_POINT('',#5891);
#1764=VERTEX_POINT('',#5898);
#1765=VERTEX_POINT('',#5900);
#1766=VERTEX_POINT('',#5902);
#1767=VERTEX_POINT('',#5907);
#1768=VERTEX_POINT('',#5909);
#1769=VERTEX_POINT('',#5911);
#1770=VERTEX_POINT('',#5915);
#1771=VERTEX_POINT('',#5919);
#1772=VERTEX_POINT('',#5920);
#1773=VERTEX_POINT('',#5923);
#1774=VERTEX_POINT('',#5925);
#1775=VERTEX_POINT('',#5927);
#1776=VERTEX_POINT('',#5931);
#1777=VERTEX_POINT('',#5933);
#1778=VERTEX_POINT('',#5935);
#1779=VERTEX_POINT('',#5940);
#1780=VERTEX_POINT('',#5942);
#1781=VERTEX_POINT('',#5944);
#1782=VERTEX_POINT('',#5946);
#1783=VERTEX_POINT('',#5948);
#1784=VERTEX_POINT('',#5950);
#1785=VERTEX_POINT('',#5980);
#1786=VERTEX_POINT('',#5982);
#1787=VERTEX_POINT('',#5984);
#1788=VERTEX_POINT('',#5986);
#1789=VERTEX_POINT('',#5988);
#1790=VERTEX_POINT('',#5990);
#1791=VERTEX_POINT('',#5994);
#1792=VERTEX_POINT('',#5999);
#1793=VERTEX_POINT('',#6000);
#1794=VERTEX_POINT('',#6003);
#1795=VERTEX_POINT('',#6005);
#1796=VERTEX_POINT('',#6007);
#1797=VERTEX_POINT('',#6011);
#1798=VERTEX_POINT('',#6013);
#1799=VERTEX_POINT('',#6015);
#1800=VERTEX_POINT('',#6017);
#1801=VERTEX_POINT('',#6019);
#1802=VERTEX_POINT('',#6021);
#1803=VERTEX_POINT('',#6025);
#1804=VERTEX_POINT('',#6030);
#1805=VERTEX_POINT('',#6031);
#1806=VERTEX_POINT('',#6034);
#1807=VERTEX_POINT('',#6036);
#1808=VERTEX_POINT('',#6038);
#1809=VERTEX_POINT('',#6042);
#1810=VERTEX_POINT('',#6044);
#1811=VERTEX_POINT('',#6048);
#1812=VERTEX_POINT('',#6057);
#1813=VERTEX_POINT('',#6058);
#1814=VERTEX_POINT('',#6060);
#1815=VERTEX_POINT('',#6062);
#1816=VERTEX_POINT('',#6064);
#1817=VERTEX_POINT('',#6066);
#1818=VERTEX_POINT('',#6071);
#1819=VERTEX_POINT('',#6075);
#1820=VERTEX_POINT('',#6076);
#1821=VERTEX_POINT('',#6086);
#1822=VERTEX_POINT('',#6087);
#1823=VERTEX_POINT('',#6089);
#1824=VERTEX_POINT('',#6091);
#1825=VERTEX_POINT('',#6093);
#1826=VERTEX_POINT('',#6095);
#1827=VERTEX_POINT('',#6100);
#1828=VERTEX_POINT('',#6104);
#1829=VERTEX_POINT('',#6105);
#1830=VERTEX_POINT('',#6115);
#1831=VERTEX_POINT('',#6116);
#1832=VERTEX_POINT('',#6118);
#1833=VERTEX_POINT('',#6120);
#1834=VERTEX_POINT('',#6122);
#1835=VERTEX_POINT('',#6124);
#1836=VERTEX_POINT('',#6129);
#1837=VERTEX_POINT('',#6133);
#1838=VERTEX_POINT('',#6134);
#1839=VERTEX_POINT('',#6144);
#1840=VERTEX_POINT('',#6145);
#1841=VERTEX_POINT('',#6147);
#1842=VERTEX_POINT('',#6149);
#1843=VERTEX_POINT('',#6151);
#1844=VERTEX_POINT('',#6153);
#1987=EDGE_CURVE('',#1641,#1642,#885,.T.);
#1988=EDGE_CURVE('',#1641,#1643,#886,.F.);
#1989=EDGE_CURVE('',#1643,#1644,#887,.T.);
#1990=EDGE_CURVE('',#1644,#1645,#888,.T.);
#1991=EDGE_CURVE('',#1646,#1645,#889,.T.);
#1992=EDGE_CURVE('',#1647,#1646,#890,.T.);
#1993=EDGE_CURVE('',#1647,#1648,#891,.T.);
#1994=EDGE_CURVE('',#1648,#1649,#892,.F.);
#1995=EDGE_CURVE('',#1650,#1649,#893,.T.);
#1996=EDGE_CURVE('',#1651,#1650,#894,.T.);
#1997=EDGE_CURVE('',#1651,#1652,#895,.T.);
#1998=EDGE_CURVE('',#1642,#1652,#896,.T.);
#1999=EDGE_CURVE('',#1653,#1653,#242,.T.);
#2000=EDGE_CURVE('',#1654,#1654,#243,.T.);
#2001=EDGE_CURVE('',#1655,#1655,#244,.T.);
#2002=EDGE_CURVE('',#1656,#1656,#245,.T.);
#2003=EDGE_CURVE('',#1657,#1658,#897,.T.);
#2004=EDGE_CURVE('',#1657,#1659,#898,.T.);
#2005=EDGE_CURVE('',#1659,#1660,#899,.T.);
#2006=EDGE_CURVE('',#1658,#1660,#900,.T.);
#2007=EDGE_CURVE('',#1661,#1662,#901,.T.);
#2008=EDGE_CURVE('',#1661,#1663,#902,.T.);
#2009=EDGE_CURVE('',#1663,#1664,#903,.T.);
#2010=EDGE_CURVE('',#1662,#1664,#904,.T.);
#2011=EDGE_CURVE('',#1665,#1666,#905,.T.);
#2012=EDGE_CURVE('',#1666,#1667,#906,.T.);
#2013=EDGE_CURVE('',#1667,#1668,#907,.T.);
#2014=EDGE_CURVE('',#1668,#1647,#908,.T.);
#2015=EDGE_CURVE('',#1646,#1669,#909,.T.);
#2016=EDGE_CURVE('',#1670,#1669,#910,.T.);
#2017=EDGE_CURVE('',#1670,#1665,#911,.T.);
#2018=EDGE_CURVE('',#1671,#1672,#912,.T.);
#2019=EDGE_CURVE('',#1672,#1673,#913,.T.);
#2020=EDGE_CURVE('',#1673,#1670,#914,.T.);
#2021=EDGE_CURVE('',#1669,#1674,#915,.T.);
#2022=EDGE_CURVE('',#1675,#1674,#916,.T.);
#2023=EDGE_CURVE('',#1675,#1676,#917,.T.);
#2024=EDGE_CURVE('',#1676,#1677,#918,.T.);
#2025=EDGE_CURVE('',#1677,#1678,#919,.T.);
#2026=EDGE_CURVE('',#1678,#1679,#920,.T.);
#2027=EDGE_CURVE('',#1679,#1680,#921,.T.);
#2028=EDGE_CURVE('',#1680,#1671,#922,.T.);
#2029=EDGE_CURVE('',#1681,#1682,#923,.T.);
#2030=EDGE_CURVE('',#1682,#1683,#924,.T.);
#2031=EDGE_CURVE('',#1683,#1675,#925,.T.);
#2032=EDGE_CURVE('',#1645,#1674,#926,.T.);
#2033=EDGE_CURVE('',#1644,#1684,#927,.T.);
#2034=EDGE_CURVE('',#1684,#1681,#928,.T.);
#2035=EDGE_CURVE('',#1685,#1686,#929,.T.);
#2036=EDGE_CURVE('',#1685,#1687,#930,.T.);
#2037=EDGE_CURVE('',#1687,#1688,#931,.T.);
#2038=EDGE_CURVE('',#1689,#1688,#932,.T.);
#2039=EDGE_CURVE('',#1690,#1689,#933,.T.);
#2040=EDGE_CURVE('',#1686,#1690,#934,.T.);
#2041=EDGE_CURVE('',#1691,#1692,#935,.T.);
#2042=EDGE_CURVE('',#1691,#1693,#936,.T.);
#2043=EDGE_CURVE('',#1694,#1693,#937,.T.);
#2044=EDGE_CURVE('',#1695,#1694,#938,.T.);
#2045=EDGE_CURVE('',#1695,#1696,#939,.T.);
#2046=EDGE_CURVE('',#1692,#1696,#940,.T.);
#2047=EDGE_CURVE('',#1697,#1698,#941,.T.);
#2048=EDGE_CURVE('',#1698,#1699,#942,.T.);
#2049=EDGE_CURVE('',#1700,#1699,#943,.T.);
#2050=EDGE_CURVE('',#1700,#1701,#944,.T.);
#2051=EDGE_CURVE('',#1701,#1702,#945,.T.);
#2052=EDGE_CURVE('',#1702,#1703,#946,.T.);
#2053=EDGE_CURVE('',#1704,#1703,#947,.T.);
#2054=EDGE_CURVE('',#1704,#1705,#948,.T.);
#2055=EDGE_CURVE('',#1705,#1706,#949,.T.);
#2056=EDGE_CURVE('',#1707,#1706,#950,.T.);
#2057=EDGE_CURVE('',#1708,#1707,#951,.T.);
#2058=EDGE_CURVE('',#1708,#1697,#952,.T.);
#2059=EDGE_CURVE('',#1709,#1710,#953,.T.);
#2060=EDGE_CURVE('',#1709,#1711,#954,.T.);
#2061=EDGE_CURVE('',#1711,#1712,#955,.T.);
#2062=EDGE_CURVE('',#1710,#1712,#956,.T.);
#2063=EDGE_CURVE('',#1713,#1713,#246,.T.);
#2064=EDGE_CURVE('',#1714,#1714,#247,.T.);
#2065=EDGE_CURVE('',#1715,#1715,#248,.T.);
#2066=EDGE_CURVE('',#1716,#1716,#249,.T.);
#2067=EDGE_CURVE('',#1717,#1718,#957,.T.);
#2068=EDGE_CURVE('',#1717,#1719,#958,.T.);
#2069=EDGE_CURVE('',#1719,#1720,#959,.T.);
#2070=EDGE_CURVE('',#1718,#1720,#960,.T.);
#2071=EDGE_CURVE('',#1721,#1722,#961,.T.);
#2072=EDGE_CURVE('',#1723,#1721,#962,.T.);
#2073=EDGE_CURVE('',#1724,#1723,#963,.T.);
#2074=EDGE_CURVE('',#1724,#1722,#964,.T.);
#2075=EDGE_CURVE('',#1725,#1699,#965,.T.);
#2076=EDGE_CURVE('',#1726,#1725,#966,.T.);
#2077=EDGE_CURVE('',#1700,#1726,#967,.T.);
#2078=EDGE_CURVE('',#1727,#1728,#968,.T.);
#2079=EDGE_CURVE('',#1704,#1727,#969,.T.);
#2080=EDGE_CURVE('',#1729,#1703,#970,.T.);
#2081=EDGE_CURVE('',#1730,#1729,#971,.T.);
#2082=EDGE_CURVE('',#1730,#1728,#972,.T.);
#2083=EDGE_CURVE('',#1731,#1732,#973,.T.);
#2084=EDGE_CURVE('',#1733,#1731,#974,.T.);
#2085=EDGE_CURVE('',#1734,#1733,#975,.T.);
#2086=EDGE_CURVE('',#1708,#1734,#976,.T.);
#2087=EDGE_CURVE('',#1707,#1732,#977,.T.);
#2088=EDGE_CURVE('',#1735,#1735,#250,.T.);
#2089=EDGE_CURVE('',#1736,#1736,#251,.T.);
#2090=EDGE_CURVE('',#1686,#1737,#978,.T.);
#2091=EDGE_CURVE('',#1690,#1738,#979,.T.);
#2092=EDGE_CURVE('',#1705,#1738,#980,.T.);
#2093=EDGE_CURVE('',#1739,#1727,#981,.T.);
#2094=EDGE_CURVE('',#1737,#1739,#982,.T.);
#2095=EDGE_CURVE('',#1740,#1721,#983,.T.);
#2096=EDGE_CURVE('',#1741,#1740,#984,.T.);
#2097=EDGE_CURVE('',#1694,#1741,#985,.T.);
#2098=EDGE_CURVE('',#1693,#1742,#986,.T.);
#2099=EDGE_CURVE('',#1738,#1742,#987,.T.);
#2100=EDGE_CURVE('',#1743,#1689,#988,.T.);
#2101=EDGE_CURVE('',#1744,#1743,#989,.T.);
#2102=EDGE_CURVE('',#1723,#1744,#990,.T.);
#2103=EDGE_CURVE('',#1691,#1745,#991,.T.);
#2104=EDGE_CURVE('',#1745,#1746,#992,.T.);
#2105=EDGE_CURVE('',#1746,#1732,#993,.T.);
#2106=EDGE_CURVE('',#1706,#1742,#994,.T.);
#2107=EDGE_CURVE('',#1747,#1747,#252,.T.);
#2108=EDGE_CURVE('',#1748,#1748,#253,.T.);
#2109=EDGE_CURVE('',#1726,#1749,#995,.T.);
#2110=EDGE_CURVE('',#1750,#1749,#996,.T.);
#2111=EDGE_CURVE('',#1751,#1750,#997,.T.);
#2112=EDGE_CURVE('',#1751,#1651,#998,.T.);
#2113=EDGE_CURVE('',#1701,#1650,#999,.T.);
#2114=EDGE_CURVE('',#1649,#1752,#254,.T.);
#2115=EDGE_CURVE('',#1702,#1752,#1000,.T.);
#2116=EDGE_CURVE('',#1752,#1753,#1001,.T.);
#2117=EDGE_CURVE('',#1754,#1753,#255,.F.);
#2118=EDGE_CURVE('',#1754,#1755,#1002,.T.);
#2119=EDGE_CURVE('',#1755,#1756,#1003,.T.);
#2120=EDGE_CURVE('',#1757,#1756,#1004,.T.);
#2121=EDGE_CURVE('',#1729,#1757,#1005,.T.);
#2122=EDGE_CURVE('',#1758,#1759,#256,.F.);
#2123=EDGE_CURVE('',#1758,#1760,#1006,.T.);
#2124=EDGE_CURVE('',#1697,#1760,#1007,.T.);
#2125=EDGE_CURVE('',#1734,#1761,#1008,.T.);
#2126=EDGE_CURVE('',#1762,#1761,#1009,.T.);
#2127=EDGE_CURVE('',#1763,#1762,#1010,.T.);
#2128=EDGE_CURVE('',#1763,#1759,#1011,.T.);
#2129=EDGE_CURVE('',#1698,#1642,#1012,.T.);
#2130=EDGE_CURVE('',#1760,#1641,#257,.T.);
#2131=EDGE_CURVE('',#1652,#1764,#1013,.T.);
#2132=EDGE_CURVE('',#1764,#1765,#1014,.T.);
#2133=EDGE_CURVE('',#1766,#1765,#1015,.T.);
#2134=EDGE_CURVE('',#1725,#1766,#1016,.T.);
#2135=EDGE_CURVE('',#1671,#1744,#1017,.T.);
#2136=EDGE_CURVE('',#1680,#1767,#1018,.T.);
#2137=EDGE_CURVE('',#1767,#1768,#1019,.T.);
#2138=EDGE_CURVE('',#1769,#1768,#1020,.T.);
#2139=EDGE_CURVE('',#1724,#1769,#1021,.T.);
#2140=EDGE_CURVE('',#1770,#1743,#1022,.T.);
#2141=EDGE_CURVE('',#1770,#1672,#258,.T.);
#2142=EDGE_CURVE('',#1771,#1772,#259,.F.);
#2143=EDGE_CURVE('',#1771,#1770,#1023,.F.);
#2144=EDGE_CURVE('',#1688,#1773,#1024,.T.);
#2145=EDGE_CURVE('',#1774,#1773,#1025,.T.);
#2146=EDGE_CURVE('',#1775,#1774,#1026,.T.);
#2147=EDGE_CURVE('',#1775,#1772,#1027,.T.);
#2148=EDGE_CURVE('',#1722,#1776,#1028,.T.);
#2149=EDGE_CURVE('',#1777,#1776,#1029,.T.);
#2150=EDGE_CURVE('',#1778,#1777,#1030,.T.);
#2151=EDGE_CURVE('',#1778,#1679,#1031,.T.);
#2152=EDGE_CURVE('',#1678,#1740,#1032,.T.);
#2153=EDGE_CURVE('',#1779,#1741,#1033,.T.);
#2154=EDGE_CURVE('',#1779,#1780,#1034,.F.);
#2155=EDGE_CURVE('',#1781,#1780,#260,.F.);
#2156=EDGE_CURVE('',#1781,#1782,#1035,.T.);
#2157=EDGE_CURVE('',#1782,#1783,#1036,.T.);
#2158=EDGE_CURVE('',#1784,#1783,#1037,.T.);
#2159=EDGE_CURVE('',#1695,#1784,#1038,.T.);
#2160=EDGE_CURVE('',#1677,#1779,#261,.T.);
#2161=EDGE_CURVE('',#1718,#1659,#1039,.T.);
#2162=EDGE_CURVE('',#1717,#1657,#1040,.T.);
#2163=EDGE_CURVE('',#1720,#1660,#1041,.T.);
#2164=EDGE_CURVE('',#1719,#1658,#1042,.T.);
#2165=EDGE_CURVE('',#1710,#1663,#1043,.T.);
#2166=EDGE_CURVE('',#1709,#1661,#1044,.T.);
#2167=EDGE_CURVE('',#1712,#1664,#1045,.T.);
#2168=EDGE_CURVE('',#1711,#1662,#1046,.T.);
#2169=EDGE_CURVE('',#1716,#1656,#1047,.T.);
#2170=EDGE_CURVE('',#1715,#1655,#1048,.T.);
#2171=EDGE_CURVE('',#1714,#1654,#1049,.T.);
#2172=EDGE_CURVE('',#1713,#1653,#1050,.T.);
#2173=EDGE_CURVE('',#1785,#1746,#1051,.T.);
#2174=EDGE_CURVE('',#1785,#1786,#1052,.F.);
#2175=EDGE_CURVE('',#1787,#1786,#262,.F.);
#2176=EDGE_CURVE('',#1787,#1788,#1053,.T.);
#2177=EDGE_CURVE('',#1788,#1789,#1054,.T.);
#2178=EDGE_CURVE('',#1790,#1789,#1055,.T.);
#2179=EDGE_CURVE('',#1731,#1790,#1056,.T.);
#2180=EDGE_CURVE('',#1791,#1745,#1057,.T.);
#2181=EDGE_CURVE('',#1791,#1682,#263,.T.);
#2182=EDGE_CURVE('',#1681,#1785,#264,.T.);
#2183=EDGE_CURVE('',#1792,#1793,#265,.F.);
#2184=EDGE_CURVE('',#1792,#1791,#1058,.F.);
#2185=EDGE_CURVE('',#1692,#1794,#1059,.T.);
#2186=EDGE_CURVE('',#1795,#1794,#1060,.T.);
#2187=EDGE_CURVE('',#1796,#1795,#1061,.T.);
#2188=EDGE_CURVE('',#1796,#1793,#1062,.T.);
#2189=EDGE_CURVE('',#1737,#1797,#1063,.T.);
#2190=EDGE_CURVE('',#1797,#1798,#1064,.F.);
#2191=EDGE_CURVE('',#1799,#1798,#266,.F.);
#2192=EDGE_CURVE('',#1799,#1800,#1065,.T.);
#2193=EDGE_CURVE('',#1800,#1801,#1066,.T.);
#2194=EDGE_CURVE('',#1802,#1801,#1067,.T.);
#2195=EDGE_CURVE('',#1685,#1802,#1068,.T.);
#2196=EDGE_CURVE('',#1739,#1803,#1069,.T.);
#2197=EDGE_CURVE('',#1803,#1667,#267,.T.);
#2198=EDGE_CURVE('',#1666,#1797,#268,.T.);
#2199=EDGE_CURVE('',#1804,#1805,#269,.F.);
#2200=EDGE_CURVE('',#1804,#1803,#1070,.F.);
#2201=EDGE_CURVE('',#1728,#1806,#1071,.T.);
#2202=EDGE_CURVE('',#1807,#1806,#1072,.T.);
#2203=EDGE_CURVE('',#1808,#1807,#1073,.T.);
#2204=EDGE_CURVE('',#1808,#1805,#1074,.T.);
#2205=EDGE_CURVE('',#1755,#1809,#1075,.T.);
#2206=EDGE_CURVE('',#1809,#1810,#1076,.T.);
#2207=EDGE_CURVE('',#1756,#1810,#1077,.T.);
#2208=EDGE_CURVE('',#1730,#1811,#1078,.T.);
#2209=EDGE_CURVE('',#1811,#1757,#1079,.T.);
#2210=EDGE_CURVE('',#1806,#1811,#1080,.T.);
#2211=EDGE_CURVE('',#1809,#1808,#1081,.T.);
#2212=EDGE_CURVE('',#1810,#1807,#1082,.T.);
#2213=EDGE_CURVE('',#1812,#1813,#1083,.F.);
#2214=EDGE_CURVE('',#1813,#1814,#1084,.F.);
#2215=EDGE_CURVE('',#1814,#1815,#1085,.F.);
#2216=EDGE_CURVE('',#1815,#1816,#1086,.F.);
#2217=EDGE_CURVE('',#1816,#1817,#1087,.F.);
#2218=EDGE_CURVE('',#1817,#1812,#1088,.F.);
#2219=EDGE_CURVE('',#1687,#1818,#1089,.T.);
#2220=EDGE_CURVE('',#1773,#1818,#1090,.T.);
#2221=EDGE_CURVE('',#1819,#1820,#1091,.T.);
#2222=EDGE_CURVE('',#1819,#1775,#1092,.T.);
#2223=EDGE_CURVE('',#1820,#1774,#1093,.T.);
#2224=EDGE_CURVE('',#1800,#1819,#1094,.T.);
#2225=EDGE_CURVE('',#1801,#1820,#1095,.T.);
#2226=EDGE_CURVE('',#1818,#1802,#1096,.T.);
#2227=EDGE_CURVE('',#1821,#1822,#1097,.F.);
#2228=EDGE_CURVE('',#1822,#1823,#1098,.F.);
#2229=EDGE_CURVE('',#1823,#1824,#1099,.F.);
#2230=EDGE_CURVE('',#1824,#1825,#1100,.F.);
#2231=EDGE_CURVE('',#1825,#1826,#1101,.F.);
#2232=EDGE_CURVE('',#1826,#1821,#1102,.F.);
#2233=EDGE_CURVE('',#1696,#1827,#1103,.T.);
#2234=EDGE_CURVE('',#1794,#1827,#1104,.T.);
#2235=EDGE_CURVE('',#1828,#1829,#1105,.T.);
#2236=EDGE_CURVE('',#1828,#1796,#1106,.T.);
#2237=EDGE_CURVE('',#1829,#1795,#1107,.T.);
#2238=EDGE_CURVE('',#1782,#1828,#1108,.T.);
#2239=EDGE_CURVE('',#1783,#1829,#1109,.T.);
#2240=EDGE_CURVE('',#1827,#1784,#1110,.T.);
#2241=EDGE_CURVE('',#1830,#1831,#1111,.F.);
#2242=EDGE_CURVE('',#1831,#1832,#1112,.F.);
#2243=EDGE_CURVE('',#1832,#1833,#1113,.F.);
#2244=EDGE_CURVE('',#1833,#1834,#1114,.F.);
#2245=EDGE_CURVE('',#1834,#1835,#1115,.F.);
#2246=EDGE_CURVE('',#1835,#1830,#1116,.F.);
#2247=EDGE_CURVE('',#1733,#1836,#1117,.T.);
#2248=EDGE_CURVE('',#1761,#1836,#1118,.T.);
#2249=EDGE_CURVE('',#1837,#1838,#1119,.T.);
#2250=EDGE_CURVE('',#1837,#1763,#1120,.T.);
#2251=EDGE_CURVE('',#1838,#1762,#1121,.T.);
#2252=EDGE_CURVE('',#1788,#1837,#1122,.T.);
#2253=EDGE_CURVE('',#1789,#1838,#1123,.T.);
#2254=EDGE_CURVE('',#1836,#1790,#1124,.T.);
#2255=EDGE_CURVE('',#1839,#1840,#1125,.F.);
#2256=EDGE_CURVE('',#1840,#1841,#1126,.F.);
#2257=EDGE_CURVE('',#1841,#1842,#1127,.F.);
#2258=EDGE_CURVE('',#1842,#1843,#1128,.F.);
#2259=EDGE_CURVE('',#1843,#1844,#1129,.F.);
#2260=EDGE_CURVE('',#1844,#1839,#1130,.F.);
#2261=EDGE_CURVE('',#1776,#1769,#1131,.T.);
#2262=EDGE_CURVE('',#1768,#1777,#1132,.T.);
#2263=EDGE_CURVE('',#1767,#1778,#1133,.T.);
#2264=EDGE_CURVE('',#1765,#1750,#1134,.T.);
#2265=EDGE_CURVE('',#1764,#1751,#1135,.T.);
#2266=EDGE_CURVE('',#1749,#1766,#1136,.T.);
#2267=EDGE_CURVE('',#1772,#1824,#270,.T.);
#2268=EDGE_CURVE('',#1825,#1775,#92,.T.);
#2269=EDGE_CURVE('',#1673,#1771,#271,.T.);
#2270=EDGE_CURVE('',#1826,#1819,#93,.F.);
#2271=EDGE_CURVE('',#1673,#1824,#272,.F.);
#2272=EDGE_CURVE('',#1821,#1800,#94,.F.);
#2273=EDGE_CURVE('',#1670,#1823,#95,.F.);
#2274=EDGE_CURVE('',#1822,#1799,#273,.T.);
#2275=EDGE_CURVE('',#1665,#1822,#274,.T.);
#2276=EDGE_CURVE('',#1665,#1798,#275,.F.);
#2277=EDGE_CURVE('',#1793,#1833,#276,.T.);
#2278=EDGE_CURVE('',#1834,#1796,#96,.F.);
#2279=EDGE_CURVE('',#1683,#1792,#277,.T.);
#2280=EDGE_CURVE('',#1835,#1828,#97,.T.);
#2281=EDGE_CURVE('',#1683,#1833,#278,.F.);
#2282=EDGE_CURVE('',#1830,#1782,#98,.T.);
#2283=EDGE_CURVE('',#1675,#1832,#99,.F.);
#2284=EDGE_CURVE('',#1831,#1781,#279,.T.);
#2285=EDGE_CURVE('',#1676,#1831,#280,.T.);
#2286=EDGE_CURVE('',#1676,#1780,#281,.F.);
#2287=EDGE_CURVE('',#1759,#1842,#282,.T.);
#2288=EDGE_CURVE('',#1843,#1763,#100,.T.);
#2289=EDGE_CURVE('',#1643,#1758,#283,.T.);
#2290=EDGE_CURVE('',#1844,#1837,#101,.F.);
#2291=EDGE_CURVE('',#1643,#1842,#284,.F.);
#2292=EDGE_CURVE('',#1839,#1788,#102,.F.);
#2293=EDGE_CURVE('',#1644,#1841,#103,.T.);
#2294=EDGE_CURVE('',#1840,#1787,#285,.T.);
#2295=EDGE_CURVE('',#1684,#1840,#286,.T.);
#2296=EDGE_CURVE('',#1684,#1786,#287,.F.);
#2297=EDGE_CURVE('',#1753,#1648,#288,.T.);
#2298=EDGE_CURVE('',#1755,#1815,#104,.F.);
#2299=EDGE_CURVE('',#1816,#1754,#289,.T.);
#2300=EDGE_CURVE('',#1816,#1648,#290,.F.);
#2301=EDGE_CURVE('',#1809,#1814,#105,.F.);
#2302=EDGE_CURVE('',#1817,#1647,#106,.T.);
#2303=EDGE_CURVE('',#1808,#1813,#107,.T.);
#2304=EDGE_CURVE('',#1812,#1668,#291,.T.);
#2305=EDGE_CURVE('',#1805,#1812,#292,.T.);
#2306=EDGE_CURVE('',#1804,#1668,#293,.F.);
#2307=EDGE_CURVE('',#1736,#1748,#1137,.T.);
#2308=EDGE_CURVE('',#1735,#1747,#1138,.T.);
#2533=ORIENTED_EDGE('',*,*,#1987,.F.);
#2534=ORIENTED_EDGE('',*,*,#1988,.T.);
#2535=ORIENTED_EDGE('',*,*,#1989,.T.);
#2536=ORIENTED_EDGE('',*,*,#1990,.T.);
#2537=ORIENTED_EDGE('',*,*,#1991,.F.);
#2538=ORIENTED_EDGE('',*,*,#1992,.F.);
#2539=ORIENTED_EDGE('',*,*,#1993,.T.);
#2540=ORIENTED_EDGE('',*,*,#1994,.T.);
#2541=ORIENTED_EDGE('',*,*,#1995,.F.);
#2542=ORIENTED_EDGE('',*,*,#1996,.F.);
#2543=ORIENTED_EDGE('',*,*,#1997,.T.);
#2544=ORIENTED_EDGE('',*,*,#1998,.F.);
#2545=ORIENTED_EDGE('',*,*,#1999,.F.);
#2546=ORIENTED_EDGE('',*,*,#2000,.F.);
#2547=ORIENTED_EDGE('',*,*,#2001,.F.);
#2548=ORIENTED_EDGE('',*,*,#2002,.F.);
#2549=ORIENTED_EDGE('',*,*,#2003,.F.);
#2550=ORIENTED_EDGE('',*,*,#2004,.T.);
#2551=ORIENTED_EDGE('',*,*,#2005,.T.);
#2552=ORIENTED_EDGE('',*,*,#2006,.F.);
#2553=ORIENTED_EDGE('',*,*,#2007,.F.);
#2554=ORIENTED_EDGE('',*,*,#2008,.T.);
#2555=ORIENTED_EDGE('',*,*,#2009,.T.);
#2556=ORIENTED_EDGE('',*,*,#2010,.F.);
#2557=ORIENTED_EDGE('',*,*,#2011,.T.);
#2558=ORIENTED_EDGE('',*,*,#2012,.T.);
#2559=ORIENTED_EDGE('',*,*,#2013,.T.);
#2560=ORIENTED_EDGE('',*,*,#2014,.T.);
#2561=ORIENTED_EDGE('',*,*,#1992,.T.);
#2562=ORIENTED_EDGE('',*,*,#2015,.T.);
#2563=ORIENTED_EDGE('',*,*,#2016,.F.);
#2564=ORIENTED_EDGE('',*,*,#2017,.T.);
#2565=ORIENTED_EDGE('',*,*,#2018,.T.);
#2566=ORIENTED_EDGE('',*,*,#2019,.T.);
#2567=ORIENTED_EDGE('',*,*,#2020,.T.);
#2568=ORIENTED_EDGE('',*,*,#2016,.T.);
#2569=ORIENTED_EDGE('',*,*,#2021,.T.);
#2570=ORIENTED_EDGE('',*,*,#2022,.F.);
#2571=ORIENTED_EDGE('',*,*,#2023,.T.);
#2572=ORIENTED_EDGE('',*,*,#2024,.T.);
#2573=ORIENTED_EDGE('',*,*,#2025,.T.);
#2574=ORIENTED_EDGE('',*,*,#2026,.T.);
#2575=ORIENTED_EDGE('',*,*,#2027,.T.);
#2576=ORIENTED_EDGE('',*,*,#2028,.T.);
#2577=ORIENTED_EDGE('',*,*,#2029,.T.);
#2578=ORIENTED_EDGE('',*,*,#2030,.T.);
#2579=ORIENTED_EDGE('',*,*,#2031,.T.);
#2580=ORIENTED_EDGE('',*,*,#2022,.T.);
#2581=ORIENTED_EDGE('',*,*,#2032,.F.);
#2582=ORIENTED_EDGE('',*,*,#1990,.F.);
#2583=ORIENTED_EDGE('',*,*,#2033,.T.);
#2584=ORIENTED_EDGE('',*,*,#2034,.T.);
#2585=ORIENTED_EDGE('',*,*,#2035,.F.);
#2586=ORIENTED_EDGE('',*,*,#2036,.T.);
#2587=ORIENTED_EDGE('',*,*,#2037,.T.);
#2588=ORIENTED_EDGE('',*,*,#2038,.F.);
#2589=ORIENTED_EDGE('',*,*,#2039,.F.);
#2590=ORIENTED_EDGE('',*,*,#2040,.F.);
#2591=ORIENTED_EDGE('',*,*,#2041,.F.);
#2592=ORIENTED_EDGE('',*,*,#2042,.T.);
#2593=ORIENTED_EDGE('',*,*,#2043,.F.);
#2594=ORIENTED_EDGE('',*,*,#2044,.F.);
#2595=ORIENTED_EDGE('',*,*,#2045,.T.);
#2596=ORIENTED_EDGE('',*,*,#2046,.F.);
#2597=ORIENTED_EDGE('',*,*,#2047,.T.);
#2598=ORIENTED_EDGE('',*,*,#2048,.T.);
#2599=ORIENTED_EDGE('',*,*,#2049,.F.);
#2600=ORIENTED_EDGE('',*,*,#2050,.T.);
#2601=ORIENTED_EDGE('',*,*,#2051,.T.);
#2602=ORIENTED_EDGE('',*,*,#2052,.T.);
#2603=ORIENTED_EDGE('',*,*,#2053,.F.);
#2604=ORIENTED_EDGE('',*,*,#2054,.T.);
#2605=ORIENTED_EDGE('',*,*,#2055,.T.);
#2606=ORIENTED_EDGE('',*,*,#2056,.F.);
#2607=ORIENTED_EDGE('',*,*,#2057,.F.);
#2608=ORIENTED_EDGE('',*,*,#2058,.T.);
#2609=ORIENTED_EDGE('',*,*,#2059,.F.);
#2610=ORIENTED_EDGE('',*,*,#2060,.T.);
#2611=ORIENTED_EDGE('',*,*,#2061,.T.);
#2612=ORIENTED_EDGE('',*,*,#2062,.F.);
#2613=ORIENTED_EDGE('',*,*,#2063,.T.);
#2614=ORIENTED_EDGE('',*,*,#2064,.T.);
#2615=ORIENTED_EDGE('',*,*,#2065,.T.);
#2616=ORIENTED_EDGE('',*,*,#2066,.T.);
#2617=ORIENTED_EDGE('',*,*,#2067,.F.);
#2618=ORIENTED_EDGE('',*,*,#2068,.T.);
#2619=ORIENTED_EDGE('',*,*,#2069,.T.);
#2620=ORIENTED_EDGE('',*,*,#2070,.F.);
#2621=ORIENTED_EDGE('',*,*,#2071,.F.);
#2622=ORIENTED_EDGE('',*,*,#2072,.F.);
#2623=ORIENTED_EDGE('',*,*,#2073,.F.);
#2624=ORIENTED_EDGE('',*,*,#2074,.T.);
#2625=ORIENTED_EDGE('',*,*,#2075,.F.);
#2626=ORIENTED_EDGE('',*,*,#2076,.F.);
#2627=ORIENTED_EDGE('',*,*,#2077,.F.);
#2628=ORIENTED_EDGE('',*,*,#2049,.T.);
#2629=ORIENTED_EDGE('',*,*,#2078,.F.);
#2630=ORIENTED_EDGE('',*,*,#2079,.F.);
#2631=ORIENTED_EDGE('',*,*,#2053,.T.);
#2632=ORIENTED_EDGE('',*,*,#2080,.F.);
#2633=ORIENTED_EDGE('',*,*,#2081,.F.);
#2634=ORIENTED_EDGE('',*,*,#2082,.T.);
#2635=ORIENTED_EDGE('',*,*,#2083,.F.);
#2636=ORIENTED_EDGE('',*,*,#2084,.F.);
#2637=ORIENTED_EDGE('',*,*,#2085,.F.);
#2638=ORIENTED_EDGE('',*,*,#2086,.F.);
#2639=ORIENTED_EDGE('',*,*,#2057,.T.);
#2640=ORIENTED_EDGE('',*,*,#2087,.T.);
#2641=ORIENTED_EDGE('',*,*,#2015,.F.);
#2642=ORIENTED_EDGE('',*,*,#1991,.T.);
#2643=ORIENTED_EDGE('',*,*,#2032,.T.);
#2644=ORIENTED_EDGE('',*,*,#2021,.F.);
#2645=ORIENTED_EDGE('',*,*,#2088,.T.);
#2646=ORIENTED_EDGE('',*,*,#2089,.T.);
#2647=ORIENTED_EDGE('',*,*,#2090,.F.);
#2648=ORIENTED_EDGE('',*,*,#2040,.T.);
#2649=ORIENTED_EDGE('',*,*,#2091,.T.);
#2650=ORIENTED_EDGE('',*,*,#2092,.F.);
#2651=ORIENTED_EDGE('',*,*,#2054,.F.);
#2652=ORIENTED_EDGE('',*,*,#2079,.T.);
#2653=ORIENTED_EDGE('',*,*,#2093,.F.);
#2654=ORIENTED_EDGE('',*,*,#2094,.F.);
#2655=ORIENTED_EDGE('',*,*,#2095,.F.);
#2656=ORIENTED_EDGE('',*,*,#2096,.F.);
#2657=ORIENTED_EDGE('',*,*,#2097,.F.);
#2658=ORIENTED_EDGE('',*,*,#2043,.T.);
#2659=ORIENTED_EDGE('',*,*,#2098,.T.);
#2660=ORIENTED_EDGE('',*,*,#2099,.F.);
#2661=ORIENTED_EDGE('',*,*,#2091,.F.);
#2662=ORIENTED_EDGE('',*,*,#2039,.T.);
#2663=ORIENTED_EDGE('',*,*,#2100,.F.);
#2664=ORIENTED_EDGE('',*,*,#2101,.F.);
#2665=ORIENTED_EDGE('',*,*,#2102,.F.);
#2666=ORIENTED_EDGE('',*,*,#2072,.T.);
#2667=ORIENTED_EDGE('',*,*,#2042,.F.);
#2668=ORIENTED_EDGE('',*,*,#2103,.T.);
#2669=ORIENTED_EDGE('',*,*,#2104,.T.);
#2670=ORIENTED_EDGE('',*,*,#2105,.T.);
#2671=ORIENTED_EDGE('',*,*,#2087,.F.);
#2672=ORIENTED_EDGE('',*,*,#2056,.T.);
#2673=ORIENTED_EDGE('',*,*,#2106,.T.);
#2674=ORIENTED_EDGE('',*,*,#2098,.F.);
#2675=ORIENTED_EDGE('',*,*,#2092,.T.);
#2676=ORIENTED_EDGE('',*,*,#2099,.T.);
#2677=ORIENTED_EDGE('',*,*,#2106,.F.);
#2678=ORIENTED_EDGE('',*,*,#2055,.F.);
#2679=ORIENTED_EDGE('',*,*,#2107,.F.);
#2680=ORIENTED_EDGE('',*,*,#2108,.F.);
#2681=ORIENTED_EDGE('',*,*,#2077,.T.);
#2682=ORIENTED_EDGE('',*,*,#2109,.T.);
#2683=ORIENTED_EDGE('',*,*,#2110,.F.);
#2684=ORIENTED_EDGE('',*,*,#2111,.F.);
#2685=ORIENTED_EDGE('',*,*,#2112,.T.);
#2686=ORIENTED_EDGE('',*,*,#1996,.T.);
#2687=ORIENTED_EDGE('',*,*,#2113,.F.);
#2688=ORIENTED_EDGE('',*,*,#2050,.F.);
#2689=ORIENTED_EDGE('',*,*,#1995,.T.);
#2690=ORIENTED_EDGE('',*,*,#2114,.T.);
#2691=ORIENTED_EDGE('',*,*,#2115,.F.);
#2692=ORIENTED_EDGE('',*,*,#2051,.F.);
#2693=ORIENTED_EDGE('',*,*,#2113,.T.);
#2694=ORIENTED_EDGE('',*,*,#2115,.T.);
#2695=ORIENTED_EDGE('',*,*,#2116,.T.);
#2696=ORIENTED_EDGE('',*,*,#2117,.F.);
#2697=ORIENTED_EDGE('',*,*,#2118,.T.);
#2698=ORIENTED_EDGE('',*,*,#2119,.T.);
#2699=ORIENTED_EDGE('',*,*,#2120,.F.);
#2700=ORIENTED_EDGE('',*,*,#2121,.F.);
#2701=ORIENTED_EDGE('',*,*,#2080,.T.);
#2702=ORIENTED_EDGE('',*,*,#2052,.F.);
#2703=ORIENTED_EDGE('',*,*,#2122,.F.);
#2704=ORIENTED_EDGE('',*,*,#2123,.T.);
#2705=ORIENTED_EDGE('',*,*,#2124,.F.);
#2706=ORIENTED_EDGE('',*,*,#2058,.F.);
#2707=ORIENTED_EDGE('',*,*,#2086,.T.);
#2708=ORIENTED_EDGE('',*,*,#2125,.T.);
#2709=ORIENTED_EDGE('',*,*,#2126,.F.);
#2710=ORIENTED_EDGE('',*,*,#2127,.F.);
#2711=ORIENTED_EDGE('',*,*,#2128,.T.);
#2712=ORIENTED_EDGE('',*,*,#1987,.T.);
#2713=ORIENTED_EDGE('',*,*,#2129,.F.);
#2714=ORIENTED_EDGE('',*,*,#2047,.F.);
#2715=ORIENTED_EDGE('',*,*,#2124,.T.);
#2716=ORIENTED_EDGE('',*,*,#2130,.T.);
#2717=ORIENTED_EDGE('',*,*,#1998,.T.);
#2718=ORIENTED_EDGE('',*,*,#2131,.T.);
#2719=ORIENTED_EDGE('',*,*,#2132,.T.);
#2720=ORIENTED_EDGE('',*,*,#2133,.F.);
#2721=ORIENTED_EDGE('',*,*,#2134,.F.);
#2722=ORIENTED_EDGE('',*,*,#2075,.T.);
#2723=ORIENTED_EDGE('',*,*,#2048,.F.);
#2724=ORIENTED_EDGE('',*,*,#2129,.T.);
#2725=ORIENTED_EDGE('',*,*,#2073,.T.);
#2726=ORIENTED_EDGE('',*,*,#2102,.T.);
#2727=ORIENTED_EDGE('',*,*,#2135,.F.);
#2728=ORIENTED_EDGE('',*,*,#2028,.F.);
#2729=ORIENTED_EDGE('',*,*,#2136,.T.);
#2730=ORIENTED_EDGE('',*,*,#2137,.T.);
#2731=ORIENTED_EDGE('',*,*,#2138,.F.);
#2732=ORIENTED_EDGE('',*,*,#2139,.F.);
#2733=ORIENTED_EDGE('',*,*,#2101,.T.);
#2734=ORIENTED_EDGE('',*,*,#2140,.F.);
#2735=ORIENTED_EDGE('',*,*,#2141,.T.);
#2736=ORIENTED_EDGE('',*,*,#2018,.F.);
#2737=ORIENTED_EDGE('',*,*,#2135,.T.);
#2738=ORIENTED_EDGE('',*,*,#2142,.F.);
#2739=ORIENTED_EDGE('',*,*,#2143,.T.);
#2740=ORIENTED_EDGE('',*,*,#2140,.T.);
#2741=ORIENTED_EDGE('',*,*,#2100,.T.);
#2742=ORIENTED_EDGE('',*,*,#2038,.T.);
#2743=ORIENTED_EDGE('',*,*,#2144,.T.);
#2744=ORIENTED_EDGE('',*,*,#2145,.F.);
#2745=ORIENTED_EDGE('',*,*,#2146,.F.);
#2746=ORIENTED_EDGE('',*,*,#2147,.T.);
#2747=ORIENTED_EDGE('',*,*,#2071,.T.);
#2748=ORIENTED_EDGE('',*,*,#2148,.T.);
#2749=ORIENTED_EDGE('',*,*,#2149,.F.);
#2750=ORIENTED_EDGE('',*,*,#2150,.F.);
#2751=ORIENTED_EDGE('',*,*,#2151,.T.);
#2752=ORIENTED_EDGE('',*,*,#2026,.F.);
#2753=ORIENTED_EDGE('',*,*,#2152,.T.);
#2754=ORIENTED_EDGE('',*,*,#2095,.T.);
#2755=ORIENTED_EDGE('',*,*,#2153,.F.);
#2756=ORIENTED_EDGE('',*,*,#2154,.T.);
#2757=ORIENTED_EDGE('',*,*,#2155,.F.);
#2758=ORIENTED_EDGE('',*,*,#2156,.T.);
#2759=ORIENTED_EDGE('',*,*,#2157,.T.);
#2760=ORIENTED_EDGE('',*,*,#2158,.F.);
#2761=ORIENTED_EDGE('',*,*,#2159,.F.);
#2762=ORIENTED_EDGE('',*,*,#2044,.T.);
#2763=ORIENTED_EDGE('',*,*,#2097,.T.);
#2764=ORIENTED_EDGE('',*,*,#2096,.T.);
#2765=ORIENTED_EDGE('',*,*,#2152,.F.);
#2766=ORIENTED_EDGE('',*,*,#2025,.F.);
#2767=ORIENTED_EDGE('',*,*,#2160,.T.);
#2768=ORIENTED_EDGE('',*,*,#2153,.T.);
#2769=ORIENTED_EDGE('',*,*,#2067,.T.);
#2770=ORIENTED_EDGE('',*,*,#2161,.T.);
#2771=ORIENTED_EDGE('',*,*,#2004,.F.);
#2772=ORIENTED_EDGE('',*,*,#2162,.F.);
#2773=ORIENTED_EDGE('',*,*,#2070,.T.);
#2774=ORIENTED_EDGE('',*,*,#2163,.T.);
#2775=ORIENTED_EDGE('',*,*,#2005,.F.);
#2776=ORIENTED_EDGE('',*,*,#2161,.F.);
#2777=ORIENTED_EDGE('',*,*,#2164,.T.);
#2778=ORIENTED_EDGE('',*,*,#2006,.T.);
#2779=ORIENTED_EDGE('',*,*,#2163,.F.);
#2780=ORIENTED_EDGE('',*,*,#2069,.F.);
#2781=ORIENTED_EDGE('',*,*,#2162,.T.);
#2782=ORIENTED_EDGE('',*,*,#2003,.T.);
#2783=ORIENTED_EDGE('',*,*,#2164,.F.);
#2784=ORIENTED_EDGE('',*,*,#2068,.F.);
#2785=ORIENTED_EDGE('',*,*,#2059,.T.);
#2786=ORIENTED_EDGE('',*,*,#2165,.T.);
#2787=ORIENTED_EDGE('',*,*,#2008,.F.);
#2788=ORIENTED_EDGE('',*,*,#2166,.F.);
#2789=ORIENTED_EDGE('',*,*,#2062,.T.);
#2790=ORIENTED_EDGE('',*,*,#2167,.T.);
#2791=ORIENTED_EDGE('',*,*,#2009,.F.);
#2792=ORIENTED_EDGE('',*,*,#2165,.F.);
#2793=ORIENTED_EDGE('',*,*,#2168,.T.);
#2794=ORIENTED_EDGE('',*,*,#2010,.T.);
#2795=ORIENTED_EDGE('',*,*,#2167,.F.);
#2796=ORIENTED_EDGE('',*,*,#2061,.F.);
#2797=ORIENTED_EDGE('',*,*,#2166,.T.);
#2798=ORIENTED_EDGE('',*,*,#2007,.T.);
#2799=ORIENTED_EDGE('',*,*,#2168,.F.);
#2800=ORIENTED_EDGE('',*,*,#2060,.F.);
#2801=ORIENTED_EDGE('',*,*,#2066,.F.);
#2802=ORIENTED_EDGE('',*,*,#2169,.T.);
#2803=ORIENTED_EDGE('',*,*,#2002,.T.);
#2804=ORIENTED_EDGE('',*,*,#2169,.F.);
#2805=ORIENTED_EDGE('',*,*,#2065,.F.);
#2806=ORIENTED_EDGE('',*,*,#2170,.T.);
#2807=ORIENTED_EDGE('',*,*,#2001,.T.);
#2808=ORIENTED_EDGE('',*,*,#2170,.F.);
#2809=ORIENTED_EDGE('',*,*,#2064,.F.);
#2810=ORIENTED_EDGE('',*,*,#2171,.T.);
#2811=ORIENTED_EDGE('',*,*,#2000,.T.);
#2812=ORIENTED_EDGE('',*,*,#2171,.F.);
#2813=ORIENTED_EDGE('',*,*,#2063,.F.);
#2814=ORIENTED_EDGE('',*,*,#2172,.T.);
#2815=ORIENTED_EDGE('',*,*,#1999,.T.);
#2816=ORIENTED_EDGE('',*,*,#2172,.F.);
#2817=ORIENTED_EDGE('',*,*,#2173,.F.);
#2818=ORIENTED_EDGE('',*,*,#2174,.T.);
#2819=ORIENTED_EDGE('',*,*,#2175,.F.);
#2820=ORIENTED_EDGE('',*,*,#2176,.T.);
#2821=ORIENTED_EDGE('',*,*,#2177,.T.);
#2822=ORIENTED_EDGE('',*,*,#2178,.F.);
#2823=ORIENTED_EDGE('',*,*,#2179,.F.);
#2824=ORIENTED_EDGE('',*,*,#2083,.T.);
#2825=ORIENTED_EDGE('',*,*,#2105,.F.);
#2826=ORIENTED_EDGE('',*,*,#2180,.F.);
#2827=ORIENTED_EDGE('',*,*,#2181,.T.);
#2828=ORIENTED_EDGE('',*,*,#2029,.F.);
#2829=ORIENTED_EDGE('',*,*,#2182,.T.);
#2830=ORIENTED_EDGE('',*,*,#2173,.T.);
#2831=ORIENTED_EDGE('',*,*,#2104,.F.);
#2832=ORIENTED_EDGE('',*,*,#2183,.F.);
#2833=ORIENTED_EDGE('',*,*,#2184,.T.);
#2834=ORIENTED_EDGE('',*,*,#2180,.T.);
#2835=ORIENTED_EDGE('',*,*,#2103,.F.);
#2836=ORIENTED_EDGE('',*,*,#2041,.T.);
#2837=ORIENTED_EDGE('',*,*,#2185,.T.);
#2838=ORIENTED_EDGE('',*,*,#2186,.F.);
#2839=ORIENTED_EDGE('',*,*,#2187,.F.);
#2840=ORIENTED_EDGE('',*,*,#2188,.T.);
#2841=ORIENTED_EDGE('',*,*,#2189,.T.);
#2842=ORIENTED_EDGE('',*,*,#2190,.T.);
#2843=ORIENTED_EDGE('',*,*,#2191,.F.);
#2844=ORIENTED_EDGE('',*,*,#2192,.T.);
#2845=ORIENTED_EDGE('',*,*,#2193,.T.);
#2846=ORIENTED_EDGE('',*,*,#2194,.F.);
#2847=ORIENTED_EDGE('',*,*,#2195,.F.);
#2848=ORIENTED_EDGE('',*,*,#2035,.T.);
#2849=ORIENTED_EDGE('',*,*,#2090,.T.);
#2850=ORIENTED_EDGE('',*,*,#2189,.F.);
#2851=ORIENTED_EDGE('',*,*,#2094,.T.);
#2852=ORIENTED_EDGE('',*,*,#2196,.T.);
#2853=ORIENTED_EDGE('',*,*,#2197,.T.);
#2854=ORIENTED_EDGE('',*,*,#2012,.F.);
#2855=ORIENTED_EDGE('',*,*,#2198,.T.);
#2856=ORIENTED_EDGE('',*,*,#2199,.F.);
#2857=ORIENTED_EDGE('',*,*,#2200,.T.);
#2858=ORIENTED_EDGE('',*,*,#2196,.F.);
#2859=ORIENTED_EDGE('',*,*,#2093,.T.);
#2860=ORIENTED_EDGE('',*,*,#2078,.T.);
#2861=ORIENTED_EDGE('',*,*,#2201,.T.);
#2862=ORIENTED_EDGE('',*,*,#2202,.F.);
#2863=ORIENTED_EDGE('',*,*,#2203,.F.);
#2864=ORIENTED_EDGE('',*,*,#2204,.T.);
#2865=ORIENTED_EDGE('',*,*,#2119,.F.);
#2866=ORIENTED_EDGE('',*,*,#2205,.T.);
#2867=ORIENTED_EDGE('',*,*,#2206,.T.);
#2868=ORIENTED_EDGE('',*,*,#2207,.F.);
#2869=ORIENTED_EDGE('',*,*,#2208,.F.);
#2870=ORIENTED_EDGE('',*,*,#2081,.T.);
#2871=ORIENTED_EDGE('',*,*,#2121,.T.);
#2872=ORIENTED_EDGE('',*,*,#2209,.F.);
#2873=ORIENTED_EDGE('',*,*,#2201,.F.);
#2874=ORIENTED_EDGE('',*,*,#2082,.F.);
#2875=ORIENTED_EDGE('',*,*,#2208,.T.);
#2876=ORIENTED_EDGE('',*,*,#2210,.F.);
#2877=ORIENTED_EDGE('',*,*,#2206,.F.);
#2878=ORIENTED_EDGE('',*,*,#2211,.T.);
#2879=ORIENTED_EDGE('',*,*,#2203,.T.);
#2880=ORIENTED_EDGE('',*,*,#2212,.F.);
#2881=ORIENTED_EDGE('',*,*,#2213,.T.);
#2882=ORIENTED_EDGE('',*,*,#2214,.T.);
#2883=ORIENTED_EDGE('',*,*,#2215,.T.);
#2884=ORIENTED_EDGE('',*,*,#2216,.T.);
#2885=ORIENTED_EDGE('',*,*,#2217,.T.);
#2886=ORIENTED_EDGE('',*,*,#2218,.T.);
#2887=ORIENTED_EDGE('',*,*,#2207,.T.);
#2888=ORIENTED_EDGE('',*,*,#2212,.T.);
#2889=ORIENTED_EDGE('',*,*,#2202,.T.);
#2890=ORIENTED_EDGE('',*,*,#2210,.T.);
#2891=ORIENTED_EDGE('',*,*,#2209,.T.);
#2892=ORIENTED_EDGE('',*,*,#2120,.T.);
#2893=ORIENTED_EDGE('',*,*,#2144,.F.);
#2894=ORIENTED_EDGE('',*,*,#2037,.F.);
#2895=ORIENTED_EDGE('',*,*,#2219,.T.);
#2896=ORIENTED_EDGE('',*,*,#2220,.F.);
#2897=ORIENTED_EDGE('',*,*,#2221,.F.);
#2898=ORIENTED_EDGE('',*,*,#2222,.T.);
#2899=ORIENTED_EDGE('',*,*,#2146,.T.);
#2900=ORIENTED_EDGE('',*,*,#2223,.F.);
#2901=ORIENTED_EDGE('',*,*,#2193,.F.);
#2902=ORIENTED_EDGE('',*,*,#2224,.T.);
#2903=ORIENTED_EDGE('',*,*,#2221,.T.);
#2904=ORIENTED_EDGE('',*,*,#2225,.F.);
#2905=ORIENTED_EDGE('',*,*,#2219,.F.);
#2906=ORIENTED_EDGE('',*,*,#2036,.F.);
#2907=ORIENTED_EDGE('',*,*,#2195,.T.);
#2908=ORIENTED_EDGE('',*,*,#2226,.F.);
#2909=ORIENTED_EDGE('',*,*,#2227,.T.);
#2910=ORIENTED_EDGE('',*,*,#2228,.T.);
#2911=ORIENTED_EDGE('',*,*,#2229,.T.);
#2912=ORIENTED_EDGE('',*,*,#2230,.T.);
#2913=ORIENTED_EDGE('',*,*,#2231,.T.);
#2914=ORIENTED_EDGE('',*,*,#2232,.T.);
#2915=ORIENTED_EDGE('',*,*,#2220,.T.);
#2916=ORIENTED_EDGE('',*,*,#2226,.T.);
#2917=ORIENTED_EDGE('',*,*,#2194,.T.);
#2918=ORIENTED_EDGE('',*,*,#2225,.T.);
#2919=ORIENTED_EDGE('',*,*,#2223,.T.);
#2920=ORIENTED_EDGE('',*,*,#2145,.T.);
#2921=ORIENTED_EDGE('',*,*,#2185,.F.);
#2922=ORIENTED_EDGE('',*,*,#2046,.T.);
#2923=ORIENTED_EDGE('',*,*,#2233,.T.);
#2924=ORIENTED_EDGE('',*,*,#2234,.F.);
#2925=ORIENTED_EDGE('',*,*,#2235,.F.);
#2926=ORIENTED_EDGE('',*,*,#2236,.T.);
#2927=ORIENTED_EDGE('',*,*,#2187,.T.);
#2928=ORIENTED_EDGE('',*,*,#2237,.F.);
#2929=ORIENTED_EDGE('',*,*,#2157,.F.);
#2930=ORIENTED_EDGE('',*,*,#2238,.T.);
#2931=ORIENTED_EDGE('',*,*,#2235,.T.);
#2932=ORIENTED_EDGE('',*,*,#2239,.F.);
#2933=ORIENTED_EDGE('',*,*,#2233,.F.);
#2934=ORIENTED_EDGE('',*,*,#2045,.F.);
#2935=ORIENTED_EDGE('',*,*,#2159,.T.);
#2936=ORIENTED_EDGE('',*,*,#2240,.F.);
#2937=ORIENTED_EDGE('',*,*,#2241,.T.);
#2938=ORIENTED_EDGE('',*,*,#2242,.T.);
#2939=ORIENTED_EDGE('',*,*,#2243,.T.);
#2940=ORIENTED_EDGE('',*,*,#2244,.T.);
#2941=ORIENTED_EDGE('',*,*,#2245,.T.);
#2942=ORIENTED_EDGE('',*,*,#2246,.T.);
#2943=ORIENTED_EDGE('',*,*,#2234,.T.);
#2944=ORIENTED_EDGE('',*,*,#2240,.T.);
#2945=ORIENTED_EDGE('',*,*,#2158,.T.);
#2946=ORIENTED_EDGE('',*,*,#2239,.T.);
#2947=ORIENTED_EDGE('',*,*,#2237,.T.);
#2948=ORIENTED_EDGE('',*,*,#2186,.T.);
#2949=ORIENTED_EDGE('',*,*,#2125,.F.);
#2950=ORIENTED_EDGE('',*,*,#2085,.T.);
#2951=ORIENTED_EDGE('',*,*,#2247,.T.);
#2952=ORIENTED_EDGE('',*,*,#2248,.F.);
#2953=ORIENTED_EDGE('',*,*,#2249,.F.);
#2954=ORIENTED_EDGE('',*,*,#2250,.T.);
#2955=ORIENTED_EDGE('',*,*,#2127,.T.);
#2956=ORIENTED_EDGE('',*,*,#2251,.F.);
#2957=ORIENTED_EDGE('',*,*,#2177,.F.);
#2958=ORIENTED_EDGE('',*,*,#2252,.T.);
#2959=ORIENTED_EDGE('',*,*,#2249,.T.);
#2960=ORIENTED_EDGE('',*,*,#2253,.F.);
#2961=ORIENTED_EDGE('',*,*,#2247,.F.);
#2962=ORIENTED_EDGE('',*,*,#2084,.T.);
#2963=ORIENTED_EDGE('',*,*,#2179,.T.);
#2964=ORIENTED_EDGE('',*,*,#2254,.F.);
#2965=ORIENTED_EDGE('',*,*,#2255,.T.);
#2966=ORIENTED_EDGE('',*,*,#2256,.T.);
#2967=ORIENTED_EDGE('',*,*,#2257,.T.);
#2968=ORIENTED_EDGE('',*,*,#2258,.T.);
#2969=ORIENTED_EDGE('',*,*,#2259,.T.);
#2970=ORIENTED_EDGE('',*,*,#2260,.T.);
#2971=ORIENTED_EDGE('',*,*,#2248,.T.);
#2972=ORIENTED_EDGE('',*,*,#2254,.T.);
#2973=ORIENTED_EDGE('',*,*,#2178,.T.);
#2974=ORIENTED_EDGE('',*,*,#2253,.T.);
#2975=ORIENTED_EDGE('',*,*,#2251,.T.);
#2976=ORIENTED_EDGE('',*,*,#2126,.T.);
#2977=ORIENTED_EDGE('',*,*,#2074,.F.);
#2978=ORIENTED_EDGE('',*,*,#2139,.T.);
#2979=ORIENTED_EDGE('',*,*,#2261,.F.);
#2980=ORIENTED_EDGE('',*,*,#2148,.F.);
#2981=ORIENTED_EDGE('',*,*,#2150,.T.);
#2982=ORIENTED_EDGE('',*,*,#2262,.F.);
#2983=ORIENTED_EDGE('',*,*,#2137,.F.);
#2984=ORIENTED_EDGE('',*,*,#2263,.T.);
#2985=ORIENTED_EDGE('',*,*,#2136,.F.);
#2986=ORIENTED_EDGE('',*,*,#2027,.F.);
#2987=ORIENTED_EDGE('',*,*,#2151,.F.);
#2988=ORIENTED_EDGE('',*,*,#2263,.F.);
#2989=ORIENTED_EDGE('',*,*,#2138,.T.);
#2990=ORIENTED_EDGE('',*,*,#2262,.T.);
#2991=ORIENTED_EDGE('',*,*,#2149,.T.);
#2992=ORIENTED_EDGE('',*,*,#2261,.T.);
#2993=ORIENTED_EDGE('',*,*,#2111,.T.);
#2994=ORIENTED_EDGE('',*,*,#2264,.F.);
#2995=ORIENTED_EDGE('',*,*,#2132,.F.);
#2996=ORIENTED_EDGE('',*,*,#2265,.T.);
#2997=ORIENTED_EDGE('',*,*,#2109,.F.);
#2998=ORIENTED_EDGE('',*,*,#2076,.T.);
#2999=ORIENTED_EDGE('',*,*,#2134,.T.);
#3000=ORIENTED_EDGE('',*,*,#2266,.F.);
#3001=ORIENTED_EDGE('',*,*,#2112,.F.);
#3002=ORIENTED_EDGE('',*,*,#2265,.F.);
#3003=ORIENTED_EDGE('',*,*,#2131,.F.);
#3004=ORIENTED_EDGE('',*,*,#1997,.F.);
#3005=ORIENTED_EDGE('',*,*,#2110,.T.);
#3006=ORIENTED_EDGE('',*,*,#2266,.T.);
#3007=ORIENTED_EDGE('',*,*,#2133,.T.);
#3008=ORIENTED_EDGE('',*,*,#2264,.T.);
#3009=ORIENTED_EDGE('',*,*,#2267,.F.);
#3010=ORIENTED_EDGE('',*,*,#2147,.F.);
#3011=ORIENTED_EDGE('',*,*,#2268,.F.);
#3012=ORIENTED_EDGE('',*,*,#2230,.F.);
#3013=ORIENTED_EDGE('',*,*,#2141,.F.);
#3014=ORIENTED_EDGE('',*,*,#2143,.F.);
#3015=ORIENTED_EDGE('',*,*,#2269,.F.);
#3016=ORIENTED_EDGE('',*,*,#2019,.F.);
#3017=ORIENTED_EDGE('',*,*,#2268,.T.);
#3018=ORIENTED_EDGE('',*,*,#2222,.F.);
#3019=ORIENTED_EDGE('',*,*,#2270,.F.);
#3020=ORIENTED_EDGE('',*,*,#2231,.F.);
#3021=ORIENTED_EDGE('',*,*,#2142,.T.);
#3022=ORIENTED_EDGE('',*,*,#2267,.T.);
#3023=ORIENTED_EDGE('',*,*,#2271,.F.);
#3024=ORIENTED_EDGE('',*,*,#2269,.T.);
#3025=ORIENTED_EDGE('',*,*,#2270,.T.);
#3026=ORIENTED_EDGE('',*,*,#2224,.F.);
#3027=ORIENTED_EDGE('',*,*,#2272,.F.);
#3028=ORIENTED_EDGE('',*,*,#2232,.F.);
#3029=ORIENTED_EDGE('',*,*,#2271,.T.);
#3030=ORIENTED_EDGE('',*,*,#2229,.F.);
#3031=ORIENTED_EDGE('',*,*,#2273,.F.);
#3032=ORIENTED_EDGE('',*,*,#2020,.F.);
#3033=ORIENTED_EDGE('',*,*,#2272,.T.);
#3034=ORIENTED_EDGE('',*,*,#2192,.F.);
#3035=ORIENTED_EDGE('',*,*,#2274,.F.);
#3036=ORIENTED_EDGE('',*,*,#2227,.F.);
#3037=ORIENTED_EDGE('',*,*,#2273,.T.);
#3038=ORIENTED_EDGE('',*,*,#2228,.F.);
#3039=ORIENTED_EDGE('',*,*,#2275,.F.);
#3040=ORIENTED_EDGE('',*,*,#2017,.F.);
#3041=ORIENTED_EDGE('',*,*,#2274,.T.);
#3042=ORIENTED_EDGE('',*,*,#2191,.T.);
#3043=ORIENTED_EDGE('',*,*,#2276,.F.);
#3044=ORIENTED_EDGE('',*,*,#2275,.T.);
#3045=ORIENTED_EDGE('',*,*,#2276,.T.);
#3046=ORIENTED_EDGE('',*,*,#2190,.F.);
#3047=ORIENTED_EDGE('',*,*,#2198,.F.);
#3048=ORIENTED_EDGE('',*,*,#2011,.F.);
#3049=ORIENTED_EDGE('',*,*,#2277,.F.);
#3050=ORIENTED_EDGE('',*,*,#2188,.F.);
#3051=ORIENTED_EDGE('',*,*,#2278,.F.);
#3052=ORIENTED_EDGE('',*,*,#2244,.F.);
#3053=ORIENTED_EDGE('',*,*,#2181,.F.);
#3054=ORIENTED_EDGE('',*,*,#2184,.F.);
#3055=ORIENTED_EDGE('',*,*,#2279,.F.);
#3056=ORIENTED_EDGE('',*,*,#2030,.F.);
#3057=ORIENTED_EDGE('',*,*,#2278,.T.);
#3058=ORIENTED_EDGE('',*,*,#2236,.F.);
#3059=ORIENTED_EDGE('',*,*,#2280,.F.);
#3060=ORIENTED_EDGE('',*,*,#2245,.F.);
#3061=ORIENTED_EDGE('',*,*,#2183,.T.);
#3062=ORIENTED_EDGE('',*,*,#2277,.T.);
#3063=ORIENTED_EDGE('',*,*,#2281,.F.);
#3064=ORIENTED_EDGE('',*,*,#2279,.T.);
#3065=ORIENTED_EDGE('',*,*,#2280,.T.);
#3066=ORIENTED_EDGE('',*,*,#2238,.F.);
#3067=ORIENTED_EDGE('',*,*,#2282,.F.);
#3068=ORIENTED_EDGE('',*,*,#2246,.F.);
#3069=ORIENTED_EDGE('',*,*,#2281,.T.);
#3070=ORIENTED_EDGE('',*,*,#2243,.F.);
#3071=ORIENTED_EDGE('',*,*,#2283,.F.);
#3072=ORIENTED_EDGE('',*,*,#2031,.F.);
#3073=ORIENTED_EDGE('',*,*,#2282,.T.);
#3074=ORIENTED_EDGE('',*,*,#2156,.F.);
#3075=ORIENTED_EDGE('',*,*,#2284,.F.);
#3076=ORIENTED_EDGE('',*,*,#2241,.F.);
#3077=ORIENTED_EDGE('',*,*,#2283,.T.);
#3078=ORIENTED_EDGE('',*,*,#2242,.F.);
#3079=ORIENTED_EDGE('',*,*,#2285,.F.);
#3080=ORIENTED_EDGE('',*,*,#2023,.F.);
#3081=ORIENTED_EDGE('',*,*,#2284,.T.);
#3082=ORIENTED_EDGE('',*,*,#2155,.T.);
#3083=ORIENTED_EDGE('',*,*,#2286,.F.);
#3084=ORIENTED_EDGE('',*,*,#2285,.T.);
#3085=ORIENTED_EDGE('',*,*,#2286,.T.);
#3086=ORIENTED_EDGE('',*,*,#2154,.F.);
#3087=ORIENTED_EDGE('',*,*,#2160,.F.);
#3088=ORIENTED_EDGE('',*,*,#2024,.F.);
#3089=ORIENTED_EDGE('',*,*,#2287,.F.);
#3090=ORIENTED_EDGE('',*,*,#2128,.F.);
#3091=ORIENTED_EDGE('',*,*,#2288,.F.);
#3092=ORIENTED_EDGE('',*,*,#2258,.F.);
#3093=ORIENTED_EDGE('',*,*,#2130,.F.);
#3094=ORIENTED_EDGE('',*,*,#2123,.F.);
#3095=ORIENTED_EDGE('',*,*,#2289,.F.);
#3096=ORIENTED_EDGE('',*,*,#1988,.F.);
#3097=ORIENTED_EDGE('',*,*,#2288,.T.);
#3098=ORIENTED_EDGE('',*,*,#2250,.F.);
#3099=ORIENTED_EDGE('',*,*,#2290,.F.);
#3100=ORIENTED_EDGE('',*,*,#2259,.F.);
#3101=ORIENTED_EDGE('',*,*,#2122,.T.);
#3102=ORIENTED_EDGE('',*,*,#2287,.T.);
#3103=ORIENTED_EDGE('',*,*,#2291,.F.);
#3104=ORIENTED_EDGE('',*,*,#2289,.T.);
#3105=ORIENTED_EDGE('',*,*,#2290,.T.);
#3106=ORIENTED_EDGE('',*,*,#2252,.F.);
#3107=ORIENTED_EDGE('',*,*,#2292,.F.);
#3108=ORIENTED_EDGE('',*,*,#2260,.F.);
#3109=ORIENTED_EDGE('',*,*,#2291,.T.);
#3110=ORIENTED_EDGE('',*,*,#2257,.F.);
#3111=ORIENTED_EDGE('',*,*,#2293,.F.);
#3112=ORIENTED_EDGE('',*,*,#1989,.F.);
#3113=ORIENTED_EDGE('',*,*,#2292,.T.);
#3114=ORIENTED_EDGE('',*,*,#2176,.F.);
#3115=ORIENTED_EDGE('',*,*,#2294,.F.);
#3116=ORIENTED_EDGE('',*,*,#2255,.F.);
#3117=ORIENTED_EDGE('',*,*,#2293,.T.);
#3118=ORIENTED_EDGE('',*,*,#2256,.F.);
#3119=ORIENTED_EDGE('',*,*,#2295,.F.);
#3120=ORIENTED_EDGE('',*,*,#2033,.F.);
#3121=ORIENTED_EDGE('',*,*,#2294,.T.);
#3122=ORIENTED_EDGE('',*,*,#2175,.T.);
#3123=ORIENTED_EDGE('',*,*,#2296,.F.);
#3124=ORIENTED_EDGE('',*,*,#2295,.T.);
#3125=ORIENTED_EDGE('',*,*,#2296,.T.);
#3126=ORIENTED_EDGE('',*,*,#2174,.F.);
#3127=ORIENTED_EDGE('',*,*,#2182,.F.);
#3128=ORIENTED_EDGE('',*,*,#2034,.F.);
#3129=ORIENTED_EDGE('',*,*,#2114,.F.);
#3130=ORIENTED_EDGE('',*,*,#1994,.F.);
#3131=ORIENTED_EDGE('',*,*,#2297,.F.);
#3132=ORIENTED_EDGE('',*,*,#2116,.F.);
#3133=ORIENTED_EDGE('',*,*,#2298,.F.);
#3134=ORIENTED_EDGE('',*,*,#2118,.F.);
#3135=ORIENTED_EDGE('',*,*,#2299,.F.);
#3136=ORIENTED_EDGE('',*,*,#2216,.F.);
#3137=ORIENTED_EDGE('',*,*,#2117,.T.);
#3138=ORIENTED_EDGE('',*,*,#2297,.T.);
#3139=ORIENTED_EDGE('',*,*,#2300,.F.);
#3140=ORIENTED_EDGE('',*,*,#2299,.T.);
#3141=ORIENTED_EDGE('',*,*,#2298,.T.);
#3142=ORIENTED_EDGE('',*,*,#2215,.F.);
#3143=ORIENTED_EDGE('',*,*,#2301,.F.);
#3144=ORIENTED_EDGE('',*,*,#2205,.F.);
#3145=ORIENTED_EDGE('',*,*,#2300,.T.);
#3146=ORIENTED_EDGE('',*,*,#1993,.F.);
#3147=ORIENTED_EDGE('',*,*,#2302,.F.);
#3148=ORIENTED_EDGE('',*,*,#2217,.F.);
#3149=ORIENTED_EDGE('',*,*,#2301,.T.);
#3150=ORIENTED_EDGE('',*,*,#2214,.F.);
#3151=ORIENTED_EDGE('',*,*,#2303,.F.);
#3152=ORIENTED_EDGE('',*,*,#2211,.F.);
#3153=ORIENTED_EDGE('',*,*,#2302,.T.);
#3154=ORIENTED_EDGE('',*,*,#2014,.F.);
#3155=ORIENTED_EDGE('',*,*,#2304,.F.);
#3156=ORIENTED_EDGE('',*,*,#2218,.F.);
#3157=ORIENTED_EDGE('',*,*,#2303,.T.);
#3158=ORIENTED_EDGE('',*,*,#2213,.F.);
#3159=ORIENTED_EDGE('',*,*,#2305,.F.);
#3160=ORIENTED_EDGE('',*,*,#2204,.F.);
#3161=ORIENTED_EDGE('',*,*,#2305,.T.);
#3162=ORIENTED_EDGE('',*,*,#2304,.T.);
#3163=ORIENTED_EDGE('',*,*,#2306,.F.);
#3164=ORIENTED_EDGE('',*,*,#2199,.T.);
#3165=ORIENTED_EDGE('',*,*,#2197,.F.);
#3166=ORIENTED_EDGE('',*,*,#2200,.F.);
#3167=ORIENTED_EDGE('',*,*,#2306,.T.);
#3168=ORIENTED_EDGE('',*,*,#2013,.F.);
#3169=ORIENTED_EDGE('',*,*,#2089,.F.);
#3170=ORIENTED_EDGE('',*,*,#2307,.T.);
#3171=ORIENTED_EDGE('',*,*,#2108,.T.);
#3172=ORIENTED_EDGE('',*,*,#2307,.F.);
#3173=ORIENTED_EDGE('',*,*,#2088,.F.);
#3174=ORIENTED_EDGE('',*,*,#2308,.T.);
#3175=ORIENTED_EDGE('',*,*,#2107,.T.);
#3176=ORIENTED_EDGE('',*,*,#2308,.F.);
#3625=PLANE('',#4037);
#3626=PLANE('',#4042);
#3627=PLANE('',#4043);
#3628=PLANE('',#4044);
#3629=PLANE('',#4045);
#3630=PLANE('',#4046);
#3631=PLANE('',#4047);
#3632=PLANE('',#4052);
#3633=PLANE('',#4053);
#3634=PLANE('',#4054);
#3635=PLANE('',#4055);
#3636=PLANE('',#4056);
#3637=PLANE('',#4059);
#3638=PLANE('',#4060);
#3639=PLANE('',#4061);
#3640=PLANE('',#4062);
#3641=PLANE('',#4065);
#3642=PLANE('',#4066);
#3643=PLANE('',#4068);
#3644=PLANE('',#4070);
#3645=PLANE('',#4072);
#3646=PLANE('',#4074);
#3647=PLANE('',#4075);
#3648=PLANE('',#4076);
#3649=PLANE('',#4078);
#3650=PLANE('',#4080);
#3651=PLANE('',#4081);
#3652=PLANE('',#4083);
#3653=PLANE('',#4085);
#3654=PLANE('',#4086);
#3655=PLANE('',#4087);
#3656=PLANE('',#4088);
#3657=PLANE('',#4089);
#3658=PLANE('',#4090);
#3659=PLANE('',#4091);
#3660=PLANE('',#4092);
#3661=PLANE('',#4097);
#3662=PLANE('',#4099);
#3663=PLANE('',#4102);
#3664=PLANE('',#4104);
#3665=PLANE('',#4106);
#3666=PLANE('',#4109);
#3667=PLANE('',#4111);
#3668=PLANE('',#4112);
#3669=PLANE('',#4113);
#3670=PLANE('',#4114);
#3671=PLANE('',#4115);
#3672=PLANE('',#4116);
#3673=PLANE('',#4117);
#3674=PLANE('',#4118);
#3675=PLANE('',#4119);
#3676=PLANE('',#4120);
#3677=PLANE('',#4121);
#3678=PLANE('',#4122);
#3679=PLANE('',#4123);
#3680=PLANE('',#4124);
#3681=PLANE('',#4125);
#3682=PLANE('',#4126);
#3683=PLANE('',#4127);
#3684=PLANE('',#4128);
#3685=PLANE('',#4129);
#3686=PLANE('',#4130);
#3687=PLANE('',#4131);
#3688=PLANE('',#4132);
#3689=PLANE('',#4133);
#3690=PLANE('',#4134);
#3691=PLANE('',#4135);
#3692=PLANE('',#4136);
#3693=PLANE('',#4137);
#3694=PLANE('',#4138);
#3695=PLANE('',#4139);
#3696=PLANE('',#4140);
#3697=PLANE('',#4141);
#3698=PLANE('',#4142);
#3744=ADVANCED_FACE('',(#394,#185,#186,#187,#188,#189,#190),#3625,.T.);
#3745=ADVANCED_FACE('',(#395),#3626,.F.);
#3746=ADVANCED_FACE('',(#396),#3627,.F.);
#3747=ADVANCED_FACE('',(#397),#3628,.T.);
#3748=ADVANCED_FACE('',(#398),#3629,.T.);
#3749=ADVANCED_FACE('',(#399),#3630,.T.);
#3750=ADVANCED_FACE('',(#400,#191,#192,#193,#194,#195,#196),#3631,.F.);
#3751=ADVANCED_FACE('',(#401),#3632,.T.);
#3752=ADVANCED_FACE('',(#402),#3633,.T.);
#3753=ADVANCED_FACE('',(#403),#3634,.T.);
#3754=ADVANCED_FACE('',(#404),#3635,.T.);
#3755=ADVANCED_FACE('',(#405,#197,#198),#3636,.F.);
#3756=ADVANCED_FACE('',(#406),#3637,.T.);
#3757=ADVANCED_FACE('',(#407),#3638,.T.);
#3758=ADVANCED_FACE('',(#408),#3639,.F.);
#3759=ADVANCED_FACE('',(#409,#199,#200),#3640,.T.);
#3760=ADVANCED_FACE('',(#410),#3641,.F.);
#3761=ADVANCED_FACE('',(#411),#3642,.F.);
#3762=ADVANCED_FACE('',(#412),#3643,.F.);
#3763=ADVANCED_FACE('',(#413),#3644,.F.);
#3764=ADVANCED_FACE('',(#414),#3645,.F.);
#3765=ADVANCED_FACE('',(#415),#3646,.F.);
#3766=ADVANCED_FACE('',(#416),#3647,.F.);
#3767=ADVANCED_FACE('',(#417),#3648,.F.);
#3768=ADVANCED_FACE('',(#418),#3649,.F.);
#3769=ADVANCED_FACE('',(#419),#3650,.F.);
#3770=ADVANCED_FACE('',(#420),#3651,.F.);
#3771=ADVANCED_FACE('',(#421),#3652,.F.);
#3772=ADVANCED_FACE('',(#422),#3653,.T.);
#3773=ADVANCED_FACE('',(#423),#3654,.T.);
#3774=ADVANCED_FACE('',(#424),#3655,.F.);
#3775=ADVANCED_FACE('',(#425),#3656,.F.);
#3776=ADVANCED_FACE('',(#426),#3657,.T.);
#3777=ADVANCED_FACE('',(#427),#3658,.T.);
#3778=ADVANCED_FACE('',(#428),#3659,.F.);
#3779=ADVANCED_FACE('',(#429),#3660,.F.);
#3780=ADVANCED_FACE('',(#430),#108,.F.);
#3781=ADVANCED_FACE('',(#431),#109,.F.);
#3782=ADVANCED_FACE('',(#432),#110,.F.);
#3783=ADVANCED_FACE('',(#433),#111,.F.);
#3784=ADVANCED_FACE('',(#434),#3661,.F.);
#3785=ADVANCED_FACE('',(#435),#3662,.F.);
#3786=ADVANCED_FACE('',(#436),#3663,.F.);
#3787=ADVANCED_FACE('',(#437),#3664,.F.);
#3788=ADVANCED_FACE('',(#438),#3665,.F.);
#3789=ADVANCED_FACE('',(#439),#3666,.F.);
#3790=ADVANCED_FACE('',(#440),#3667,.T.);
#3791=ADVANCED_FACE('',(#441),#3668,.T.);
#3792=ADVANCED_FACE('',(#442),#3669,.T.);
#3793=ADVANCED_FACE('',(#443),#3670,.T.);
#3794=ADVANCED_FACE('',(#444),#3671,.F.);
#3795=ADVANCED_FACE('',(#445),#3672,.T.);
#3796=ADVANCED_FACE('',(#446),#3673,.T.);
#3797=ADVANCED_FACE('',(#447),#3674,.T.);
#3798=ADVANCED_FACE('',(#448),#3675,.T.);
#3799=ADVANCED_FACE('',(#449),#3676,.T.);
#3800=ADVANCED_FACE('',(#450),#3677,.T.);
#3801=ADVANCED_FACE('',(#451),#3678,.F.);
#3802=ADVANCED_FACE('',(#452),#3679,.T.);
#3803=ADVANCED_FACE('',(#453),#3680,.T.);
#3804=ADVANCED_FACE('',(#454),#3681,.T.);
#3805=ADVANCED_FACE('',(#455),#3682,.T.);
#3806=ADVANCED_FACE('',(#456),#3683,.F.);
#3807=ADVANCED_FACE('',(#457),#3684,.T.);
#3808=ADVANCED_FACE('',(#458),#3685,.T.);
#3809=ADVANCED_FACE('',(#459),#3686,.T.);
#3810=ADVANCED_FACE('',(#460),#3687,.T.);
#3811=ADVANCED_FACE('',(#461),#3688,.T.);
#3812=ADVANCED_FACE('',(#462),#3689,.T.);
#3813=ADVANCED_FACE('',(#463),#3690,.F.);
#3814=ADVANCED_FACE('',(#464),#3691,.T.);
#3815=ADVANCED_FACE('',(#465),#3692,.T.);
#3816=ADVANCED_FACE('',(#466),#3693,.F.);
#3817=ADVANCED_FACE('',(#467),#3694,.T.);
#3818=ADVANCED_FACE('',(#468),#3695,.T.);
#3819=ADVANCED_FACE('',(#469),#3696,.T.);
#3820=ADVANCED_FACE('',(#470),#3697,.T.);
#3821=ADVANCED_FACE('',(#471),#3698,.F.);
#3822=ADVANCED_FACE('',(#472),#112,.T.);
#3823=ADVANCED_FACE('',(#473),#113,.T.);
#3824=ADVANCED_FACE('',(#474),#114,.T.);
#3825=ADVANCED_FACE('',(#475),#78,.T.);
#3826=ADVANCED_FACE('',(#476),#115,.T.);
#3827=ADVANCED_FACE('',(#477),#116,.F.);
#3828=ADVANCED_FACE('',(#478),#117,.T.);
#3829=ADVANCED_FACE('',(#479),#118,.F.);
#3830=ADVANCED_FACE('',(#480),#79,.T.);
#3831=ADVANCED_FACE('',(#481),#119,.T.);
#3832=ADVANCED_FACE('',(#482),#120,.T.);
#3833=ADVANCED_FACE('',(#483),#121,.T.);
#3834=ADVANCED_FACE('',(#484),#122,.T.);
#3835=ADVANCED_FACE('',(#485),#80,.T.);
#3836=ADVANCED_FACE('',(#486),#123,.T.);
#3837=ADVANCED_FACE('',(#487),#124,.F.);
#3838=ADVANCED_FACE('',(#488),#125,.T.);
#3839=ADVANCED_FACE('',(#489),#126,.F.);
#3840=ADVANCED_FACE('',(#490),#81,.T.);
#3841=ADVANCED_FACE('',(#491),#127,.T.);
#3842=ADVANCED_FACE('',(#492),#128,.T.);
#3843=ADVANCED_FACE('',(#493),#129,.T.);
#3844=ADVANCED_FACE('',(#494),#130,.T.);
#3845=ADVANCED_FACE('',(#495),#82,.T.);
#3846=ADVANCED_FACE('',(#496),#131,.T.);
#3847=ADVANCED_FACE('',(#497),#132,.F.);
#3848=ADVANCED_FACE('',(#498),#133,.T.);
#3849=ADVANCED_FACE('',(#499),#134,.F.);
#3850=ADVANCED_FACE('',(#500),#83,.T.);
#3851=ADVANCED_FACE('',(#501),#135,.T.);
#3852=ADVANCED_FACE('',(#502),#136,.T.);
#3853=ADVANCED_FACE('',(#503),#137,.T.);
#3854=ADVANCED_FACE('',(#504),#84,.T.);
#3855=ADVANCED_FACE('',(#505),#138,.T.);
#3856=ADVANCED_FACE('',(#506),#139,.F.);
#3857=ADVANCED_FACE('',(#507),#140,.T.);
#3858=ADVANCED_FACE('',(#508),#141,.F.);
#3859=ADVANCED_FACE('',(#509),#142,.T.);
#3860=ADVANCED_FACE('',(#510),#85,.T.);
#3861=ADVANCED_FACE('',(#511),#143,.T.);
#3862=ADVANCED_FACE('',(#512),#144,.F.);
#3863=ADVANCED_FACE('',(#513),#145,.F.);
#3961=CLOSED_SHELL('',(#3744,#3745,#3746,#3747,#3748,#3749,#3750,#3751,
#3752,#3753,#3754,#3755,#3756,#3757,#3758,#3759,#3760,#3761,#3762,#3763,
#3764,#3765,#3766,#3767,#3768,#3769,#3770,#3771,#3772,#3773,#3774,#3775,
#3776,#3777,#3778,#3779,#3780,#3781,#3782,#3783,#3784,#3785,#3786,#3787,
#3788,#3789,#3790,#3791,#3792,#3793,#3794,#3795,#3796,#3797,#3798,#3799,
#3800,#3801,#3802,#3803,#3804,#3805,#3806,#3807,#3808,#3809,#3810,#3811,
#3812,#3813,#3814,#3815,#3816,#3817,#3818,#3819,#3820,#3821,#3822,#3823,
#3824,#3825,#3826,#3827,#3828,#3829,#3830,#3831,#3832,#3833,#3834,#3835,
#3836,#3837,#3838,#3839,#3840,#3841,#3842,#3843,#3844,#3845,#3846,#3847,
#3848,#3849,#3850,#3851,#3852,#3853,#3854,#3855,#3856,#3857,#3858,#3859,
#3860,#3861,#3862,#3863));
#4036=AXIS2_PLACEMENT_3D('',#5608,#4436,#4437);
#4037=AXIS2_PLACEMENT_3D('',#5609,#4438,#4439);
#4038=AXIS2_PLACEMENT_3D('',#5635,#4452,#4453);
#4039=AXIS2_PLACEMENT_3D('',#5637,#4454,#4455);
#4040=AXIS2_PLACEMENT_3D('',#5639,#4456,#4457);
#4041=AXIS2_PLACEMENT_3D('',#5641,#4458,#4459);
#4042=AXIS2_PLACEMENT_3D('',#5658,#4468,#4469);
#4043=AXIS2_PLACEMENT_3D('',#5672,#4477,#4478);
#4044=AXIS2_PLACEMENT_3D('',#5694,#4490,#4491);
#4045=AXIS2_PLACEMENT_3D('',#5705,#4498,#4499);
#4046=AXIS2_PLACEMENT_3D('',#5718,#4506,#4507);
#4047=AXIS2_PLACEMENT_3D('',#5731,#4514,#4515);
#4048=AXIS2_PLACEMENT_3D('',#5765,#4532,#4533);
#4049=AXIS2_PLACEMENT_3D('',#5767,#4534,#4535);
#4050=AXIS2_PLACEMENT_3D('',#5769,#4536,#4537);
#4051=AXIS2_PLACEMENT_3D('',#5771,#4538,#4539);
#4052=AXIS2_PLACEMENT_3D('',#5780,#4544,#4545);
#4053=AXIS2_PLACEMENT_3D('',#5789,#4550,#4551);
#4054=AXIS2_PLACEMENT_3D('',#5795,#4555,#4556);
#4055=AXIS2_PLACEMENT_3D('',#5805,#4562,#4563);
#4056=AXIS2_PLACEMENT_3D('',#5815,#4569,#4570);
#4057=AXIS2_PLACEMENT_3D('',#5817,#4571,#4572);
#4058=AXIS2_PLACEMENT_3D('',#5819,#4573,#4574);
#4059=AXIS2_PLACEMENT_3D('',#5820,#4575,#4576);
#4060=AXIS2_PLACEMENT_3D('',#5829,#4582,#4583);
#4061=AXIS2_PLACEMENT_3D('',#5843,#4592,#4593);
#4062=AXIS2_PLACEMENT_3D('',#5850,#4598,#4599);
#4063=AXIS2_PLACEMENT_3D('',#5852,#4600,#4601);
#4064=AXIS2_PLACEMENT_3D('',#5854,#4602,#4603);
#4065=AXIS2_PLACEMENT_3D('',#5855,#4604,#4605);
#4066=AXIS2_PLACEMENT_3D('',#5864,#4611,#4612);
#4067=AXIS2_PLACEMENT_3D('',#5866,#4613,#4614);
#4068=AXIS2_PLACEMENT_3D('',#5868,#4616,#4617);
#4069=AXIS2_PLACEMENT_3D('',#5872,#4619,#4620);
#4070=AXIS2_PLACEMENT_3D('',#5880,#4625,#4626);
#4071=AXIS2_PLACEMENT_3D('',#5883,#4627,#4628);
#4072=AXIS2_PLACEMENT_3D('',#5894,#4635,#4636);
#4073=AXIS2_PLACEMENT_3D('',#5896,#4638,#4639);
#4074=AXIS2_PLACEMENT_3D('',#5897,#4640,#4641);
#4075=AXIS2_PLACEMENT_3D('',#5905,#4646,#4647);
#4076=AXIS2_PLACEMENT_3D('',#5914,#4653,#4654);
#4077=AXIS2_PLACEMENT_3D('',#5917,#4656,#4657);
#4078=AXIS2_PLACEMENT_3D('',#5918,#4658,#4659);
#4079=AXIS2_PLACEMENT_3D('',#5921,#4660,#4661);
#4080=AXIS2_PLACEMENT_3D('',#5930,#4667,#4668);
#4081=AXIS2_PLACEMENT_3D('',#5939,#4674,#4675);
#4082=AXIS2_PLACEMENT_3D('',#5945,#4678,#4679);
#4083=AXIS2_PLACEMENT_3D('',#5953,#4684,#4685);
#4084=AXIS2_PLACEMENT_3D('',#5954,#4686,#4687);
#4085=AXIS2_PLACEMENT_3D('',#5955,#4688,#4689);
#4086=AXIS2_PLACEMENT_3D('',#5958,#4692,#4693);
#4087=AXIS2_PLACEMENT_3D('',#5960,#4695,#4696);
#4088=AXIS2_PLACEMENT_3D('',#5962,#4698,#4699);
#4089=AXIS2_PLACEMENT_3D('',#5963,#4700,#4701);
#4090=AXIS2_PLACEMENT_3D('',#5966,#4704,#4705);
#4091=AXIS2_PLACEMENT_3D('',#5968,#4707,#4708);
#4092=AXIS2_PLACEMENT_3D('',#5970,#4710,#4711);
#4093=AXIS2_PLACEMENT_3D('',#5971,#4712,#4713);
#4094=AXIS2_PLACEMENT_3D('',#5973,#4715,#4716);
#4095=AXIS2_PLACEMENT_3D('',#5975,#4718,#4719);
#4096=AXIS2_PLACEMENT_3D('',#5977,#4721,#4722);
#4097=AXIS2_PLACEMENT_3D('',#5979,#4724,#4725);
#4098=AXIS2_PLACEMENT_3D('',#5985,#4728,#4729);
#4099=AXIS2_PLACEMENT_3D('',#5993,#4734,#4735);
#4100=AXIS2_PLACEMENT_3D('',#5996,#4737,#4738);
#4101=AXIS2_PLACEMENT_3D('',#5997,#4739,#4740);
#4102=AXIS2_PLACEMENT_3D('',#5998,#4741,#4742);
#4103=AXIS2_PLACEMENT_3D('',#6001,#4743,#4744);
#4104=AXIS2_PLACEMENT_3D('',#6010,#4750,#4751);
#4105=AXIS2_PLACEMENT_3D('',#6016,#4754,#4755);
#4106=AXIS2_PLACEMENT_3D('',#6024,#4760,#4761);
#4107=AXIS2_PLACEMENT_3D('',#6027,#4763,#4764);
#4108=AXIS2_PLACEMENT_3D('',#6028,#4765,#4766);
#4109=AXIS2_PLACEMENT_3D('',#6029,#4767,#4768);
#4110=AXIS2_PLACEMENT_3D('',#6032,#4769,#4770);
#4111=AXIS2_PLACEMENT_3D('',#6041,#4776,#4777);
#4112=AXIS2_PLACEMENT_3D('',#6047,#4781,#4782);
#4113=AXIS2_PLACEMENT_3D('',#6051,#4785,#4786);
#4114=AXIS2_PLACEMENT_3D('',#6053,#4788,#4789);
#4115=AXIS2_PLACEMENT_3D('',#6056,#4792,#4793);
#4116=AXIS2_PLACEMENT_3D('',#6069,#4800,#4801);
#4117=AXIS2_PLACEMENT_3D('',#6070,#4802,#4803);
#4118=AXIS2_PLACEMENT_3D('',#6074,#4806,#4807);
#4119=AXIS2_PLACEMENT_3D('',#6080,#4811,#4812);
#4120=AXIS2_PLACEMENT_3D('',#6083,#4815,#4816);
#4121=AXIS2_PLACEMENT_3D('',#6085,#4818,#4819);
#4122=AXIS2_PLACEMENT_3D('',#6098,#4826,#4827);
#4123=AXIS2_PLACEMENT_3D('',#6099,#4828,#4829);
#4124=AXIS2_PLACEMENT_3D('',#6103,#4832,#4833);
#4125=AXIS2_PLACEMENT_3D('',#6109,#4837,#4838);
#4126=AXIS2_PLACEMENT_3D('',#6112,#4841,#4842);
#4127=AXIS2_PLACEMENT_3D('',#6114,#4844,#4845);
#4128=AXIS2_PLACEMENT_3D('',#6127,#4852,#4853);
#4129=AXIS2_PLACEMENT_3D('',#6128,#4854,#4855);
#4130=AXIS2_PLACEMENT_3D('',#6132,#4858,#4859);
#4131=AXIS2_PLACEMENT_3D('',#6138,#4863,#4864);
#4132=AXIS2_PLACEMENT_3D('',#6141,#4867,#4868);
#4133=AXIS2_PLACEMENT_3D('',#6143,#4870,#4871);
#4134=AXIS2_PLACEMENT_3D('',#6156,#4878,#4879);
#4135=AXIS2_PLACEMENT_3D('',#6157,#4880,#4881);
#4136=AXIS2_PLACEMENT_3D('',#6159,#4883,#4884);
#4137=AXIS2_PLACEMENT_3D('',#6162,#4887,#4888);
#4138=AXIS2_PLACEMENT_3D('',#6163,#4889,#4890);
#4139=AXIS2_PLACEMENT_3D('',#6164,#4891,#4892);
#4140=AXIS2_PLACEMENT_3D('',#6167,#4895,#4896);
#4141=AXIS2_PLACEMENT_3D('',#6169,#4898,#4899);
#4142=AXIS2_PLACEMENT_3D('',#6170,#4900,#4901);
#4143=AXIS2_PLACEMENT_3D('',#6171,#4902,#4903);
#4144=AXIS2_PLACEMENT_3D('',#6172,#4904,#4905);
#4145=AXIS2_PLACEMENT_3D('',#6173,#4906,#4907);
#4146=AXIS2_PLACEMENT_3D('',#6174,#4908,#4909);
#4147=AXIS2_PLACEMENT_3D('',#6175,#4910,#4911);
#4148=AXIS2_PLACEMENT_3D('',#6176,#4912,#4913);
#4149=AXIS2_PLACEMENT_3D('',#6177,#4914,#4915);
#4150=AXIS2_PLACEMENT_3D('',#6178,#4916,#4917);
#4151=AXIS2_PLACEMENT_3D('',#6179,#4918,#4919);
#4152=AXIS2_PLACEMENT_3D('',#6180,#4920,#4921);
#4153=AXIS2_PLACEMENT_3D('',#6181,#4922,#4923);
#4154=AXIS2_PLACEMENT_3D('',#6182,#4924,#4925);
#4155=AXIS2_PLACEMENT_3D('',#6183,#4926,#4927);
#4156=AXIS2_PLACEMENT_3D('',#6184,#4928,#4929);
#4157=AXIS2_PLACEMENT_3D('',#6185,#4930,#4931);
#4158=AXIS2_PLACEMENT_3D('',#6186,#4932,#4933);
#4159=AXIS2_PLACEMENT_3D('',#6187,#4934,#4935);
#4160=AXIS2_PLACEMENT_3D('',#6188,#4936,#4937);
#4161=AXIS2_PLACEMENT_3D('',#6189,#4938,#4939);
#4162=AXIS2_PLACEMENT_3D('',#6190,#4940,#4941);
#4163=AXIS2_PLACEMENT_3D('',#6191,#4942,#4943);
#4164=AXIS2_PLACEMENT_3D('',#6192,#4944,#4945);
#4165=AXIS2_PLACEMENT_3D('',#6193,#4946,#4947);
#4166=AXIS2_PLACEMENT_3D('',#6194,#4948,#4949);
#4167=AXIS2_PLACEMENT_3D('',#6195,#4950,#4951);
#4168=AXIS2_PLACEMENT_3D('',#6196,#4952,#4953);
#4169=AXIS2_PLACEMENT_3D('',#6197,#4954,#4955);
#4170=AXIS2_PLACEMENT_3D('',#6198,#4956,#4957);
#4171=AXIS2_PLACEMENT_3D('',#6199,#4958,#4959);
#4172=AXIS2_PLACEMENT_3D('',#6200,#4960,#4961);
#4173=AXIS2_PLACEMENT_3D('',#6201,#4962,#4963);
#4174=AXIS2_PLACEMENT_3D('',#6202,#4964,#4965);
#4175=AXIS2_PLACEMENT_3D('',#6203,#4966,#4967);
#4176=AXIS2_PLACEMENT_3D('',#6204,#4968,#4969);
#4177=AXIS2_PLACEMENT_3D('',#6205,#4970,#4971);
#4178=AXIS2_PLACEMENT_3D('',#6206,#4972,#4973);
#4179=AXIS2_PLACEMENT_3D('',#6207,#4974,#4975);
#4180=AXIS2_PLACEMENT_3D('',#6208,#4976,#4977);
#4181=AXIS2_PLACEMENT_3D('',#6209,#4978,#4979);
#4182=AXIS2_PLACEMENT_3D('',#6210,#4980,#4981);
#4183=AXIS2_PLACEMENT_3D('',#6211,#4982,#4983);
#4184=AXIS2_PLACEMENT_3D('',#6212,#4984,#4985);
#4185=AXIS2_PLACEMENT_3D('',#6213,#4986,#4987);
#4186=AXIS2_PLACEMENT_3D('',#6214,#4988,#4989);
#4187=AXIS2_PLACEMENT_3D('',#6215,#4990,#4991);
#4188=AXIS2_PLACEMENT_3D('',#6216,#4992,#4993);
#4189=AXIS2_PLACEMENT_3D('',#6217,#4994,#4995);
#4190=AXIS2_PLACEMENT_3D('',#6218,#4996,#4997);
#4191=AXIS2_PLACEMENT_3D('',#6219,#4998,#4999);
#4192=AXIS2_PLACEMENT_3D('',#6220,#5000,#5001);
#4193=AXIS2_PLACEMENT_3D('',#6221,#5002,#5003);
#4194=AXIS2_PLACEMENT_3D('',#6222,#5004,#5005);
#4195=AXIS2_PLACEMENT_3D('',#6223,#5006,#5007);
#4196=AXIS2_PLACEMENT_3D('',#6224,#5008,#5009);
#4197=AXIS2_PLACEMENT_3D('',#6225,#5010,#5011);
#4198=AXIS2_PLACEMENT_3D('',#6226,#5012,#5013);
#4199=AXIS2_PLACEMENT_3D('',#6227,#5014,#5015);
#4200=AXIS2_PLACEMENT_3D('',#6228,#5016,#5017);
#4201=AXIS2_PLACEMENT_3D('',#6229,#5018,#5019);
#4202=AXIS2_PLACEMENT_3D('',#6230,#5020,#5021);
#4203=AXIS2_PLACEMENT_3D('',#6231,#5022,#5023);
#4204=AXIS2_PLACEMENT_3D('',#6232,#5024,#5025);
#4205=AXIS2_PLACEMENT_3D('',#6233,#5026,#5027);
#4206=AXIS2_PLACEMENT_3D('',#6234,#5028,#5029);
#4207=AXIS2_PLACEMENT_3D('',#6235,#5030,#5031);
#4208=AXIS2_PLACEMENT_3D('',#6236,#5032,#5033);
#4209=AXIS2_PLACEMENT_3D('',#6237,#5034,#5035);
#4210=AXIS2_PLACEMENT_3D('',#6238,#5036,#5037);
#4211=AXIS2_PLACEMENT_3D('',#6239,#5038,#5039);
#4212=AXIS2_PLACEMENT_3D('',#6240,#5040,#5041);
#4213=AXIS2_PLACEMENT_3D('',#6241,#5042,#5043);
#4214=AXIS2_PLACEMENT_3D('',#6242,#5044,#5045);
#4215=AXIS2_PLACEMENT_3D('',#6243,#5046,#5047);
#4216=AXIS2_PLACEMENT_3D('',#6244,#5048,#5049);
#4217=AXIS2_PLACEMENT_3D('',#6245,#5050,#5051);
#4218=AXIS2_PLACEMENT_3D('',#6246,#5052,#5053);
#4219=AXIS2_PLACEMENT_3D('',#6247,#5054,#5055);
#4220=AXIS2_PLACEMENT_3D('',#6248,#5056,#5057);
#4221=AXIS2_PLACEMENT_3D('',#6249,#5058,#5059);
#4222=AXIS2_PLACEMENT_3D('',#6250,#5060,#5061);
#4223=AXIS2_PLACEMENT_3D('',#6251,#5062,#5063);
#4224=AXIS2_PLACEMENT_3D('',#6253,#5065,#5066);
#4436=DIRECTION('axis',(0.,0.,1.));
#4437=DIRECTION('refdir',(1.,0.,0.));
#4438=DIRECTION('center_axis',(0.,0.,1.));
#4439=DIRECTION('ref_axis',(1.,0.,0.));
#4440=DIRECTION('',(-1.,0.,0.));
#4441=DIRECTION('',(0.,1.,0.));
#4442=DIRECTION('',(1.,0.,0.));
#4443=DIRECTION('',(0.,1.,0.));
#4444=DIRECTION('',(1.,0.,0.));
#4445=DIRECTION('',(0.,1.,0.));
#4446=DIRECTION('',(1.,0.,0.));
#4447=DIRECTION('',(0.,-1.,0.));
#4448=DIRECTION('',(-1.,0.,0.));
#4449=DIRECTION('',(0.,1.,0.));
#4450=DIRECTION('',(1.,0.,0.));
#4451=DIRECTION('',(0.,-1.,0.));
#4452=DIRECTION('center_axis',(0.,0.,1.));
#4453=DIRECTION('ref_axis',(1.,0.,0.));
#4454=DIRECTION('center_axis',(0.,0.,1.));
#4455=DIRECTION('ref_axis',(1.,0.,0.));
#4456=DIRECTION('center_axis',(0.,0.,1.));
#4457=DIRECTION('ref_axis',(1.,0.,0.));
#4458=DIRECTION('center_axis',(0.,0.,1.));
#4459=DIRECTION('ref_axis',(1.,0.,0.));
#4460=DIRECTION('',(1.14603667058081E-16,-1.,0.));
#4461=DIRECTION('',(1.,0.,0.));
#4462=DIRECTION('',(-2.29207334116161E-16,-1.,0.));
#4463=DIRECTION('',(1.,0.,0.));
#4464=DIRECTION('',(-1.,0.,0.));
#4465=DIRECTION('',(0.,-1.,0.));
#4466=DIRECTION('',(-1.,0.,0.));
#4467=DIRECTION('',(0.,-1.,0.));
#4468=DIRECTION('center_axis',(1.,0.,1.85037170770859E-16));
#4469=DIRECTION('ref_axis',(1.85037170770859E-16,0.,-1.));
#4470=DIRECTION('',(0.,1.,0.));
#4471=DIRECTION('',(-2.83084755282908E-16,2.83084755282908E-16,1.));
#4472=DIRECTION('',(0.,-1.,0.));
#4473=DIRECTION('',(0.,0.,1.));
#4474=DIRECTION('',(2.368475785867E-16,0.,-1.));
#4475=DIRECTION('',(0.,1.,0.));
#4476=DIRECTION('',(0.,0.,1.));
#4477=DIRECTION('center_axis',(0.,0.,1.));
#4478=DIRECTION('ref_axis',(1.,0.,0.));
#4479=DIRECTION('',(-1.,0.,0.));
#4480=DIRECTION('',(0.,-1.,0.));
#4481=DIRECTION('',(-1.,0.,0.));
#4482=DIRECTION('',(1.,0.,0.));
#4483=DIRECTION('',(0.,1.,0.));
#4484=DIRECTION('',(-1.,0.,0.));
#4485=DIRECTION('',(0.,1.,0.));
#4486=DIRECTION('',(-1.,0.,0.));
#4487=DIRECTION('',(0.,-1.,0.));
#4488=DIRECTION('',(-1.,0.,0.));
#4489=DIRECTION('',(0.,1.,0.));
#4490=DIRECTION('center_axis',(1.,0.,0.));
#4491=DIRECTION('ref_axis',(0.,0.,-1.));
#4492=DIRECTION('',(0.,-2.83084755282908E-16,-1.));
#4493=DIRECTION('',(0.,-1.,0.));
#4494=DIRECTION('',(0.,0.,-1.));
#4495=DIRECTION('',(0.,0.,-1.));
#4496=DIRECTION('',(0.,0.,-1.));
#4497=DIRECTION('',(0.,1.,0.));
#4498=DIRECTION('center_axis',(0.,-1.,0.));
#4499=DIRECTION('ref_axis',(0.,0.,-1.));
#4500=DIRECTION('',(1.,0.,0.));
#4501=DIRECTION('',(0.,0.,-1.));
#4502=DIRECTION('',(1.,0.,0.));
#4503=DIRECTION('',(0.,0.,-1.));
#4504=DIRECTION('',(1.,0.,0.));
#4505=DIRECTION('',(0.,0.,-1.));
#4506=DIRECTION('center_axis',(0.,-1.,0.));
#4507=DIRECTION('ref_axis',(0.,0.,-1.));
#4508=DIRECTION('',(1.,0.,0.));
#4509=DIRECTION('',(0.,0.,-1.));
#4510=DIRECTION('',(1.,0.,0.));
#4511=DIRECTION('',(0.,0.,1.));
#4512=DIRECTION('',(1.,0.,0.));
#4513=DIRECTION('',(0.,0.,-1.));
#4514=DIRECTION('center_axis',(0.,0.,1.));
#4515=DIRECTION('ref_axis',(1.,0.,0.));
#4516=DIRECTION('',(-1.,0.,0.));
#4517=DIRECTION('',(0.,-1.,0.));
#4518=DIRECTION('',(1.,0.,0.));
#4519=DIRECTION('',(0.,1.,0.));
#4520=DIRECTION('',(-1.,0.,0.));
#4521=DIRECTION('',(0.,-1.,0.));
#4522=DIRECTION('',(1.,0.,0.));
#4523=DIRECTION('',(0.,1.,0.));
#4524=DIRECTION('',(1.,0.,0.));
#4525=DIRECTION('',(0.,1.,0.));
#4526=DIRECTION('',(1.,0.,0.));
#4527=DIRECTION('',(0.,1.,0.));
#4528=DIRECTION('',(0.,-1.,0.));
#4529=DIRECTION('',(-1.,0.,0.));
#4530=DIRECTION('',(0.,-1.,0.));
#4531=DIRECTION('',(-1.,0.,0.));
#4532=DIRECTION('center_axis',(0.,0.,1.));
#4533=DIRECTION('ref_axis',(1.,0.,0.));
#4534=DIRECTION('center_axis',(0.,0.,1.));
#4535=DIRECTION('ref_axis',(1.,0.,0.));
#4536=DIRECTION('center_axis',(0.,0.,1.));
#4537=DIRECTION('ref_axis',(1.,0.,0.));
#4538=DIRECTION('center_axis',(0.,0.,1.));
#4539=DIRECTION('ref_axis',(1.,0.,0.));
#4540=DIRECTION('',(1.,0.,0.));
#4541=DIRECTION('',(1.14603667058081E-16,-1.,0.));
#4542=DIRECTION('',(1.,0.,0.));
#4543=DIRECTION('',(-2.29207334116161E-16,-1.,0.));
#4544=DIRECTION('center_axis',(0.,-1.,0.));
#4545=DIRECTION('ref_axis',(0.,0.,-1.));
#4546=DIRECTION('',(0.,0.,-1.));
#4547=DIRECTION('',(1.,0.,0.));
#4548=DIRECTION('',(0.,0.,1.));
#4549=DIRECTION('',(1.,0.,0.));
#4550=DIRECTION('center_axis',(0.,-1.,0.));
#4551=DIRECTION('ref_axis',(0.,0.,-1.));
#4552=DIRECTION('',(0.,0.,-1.));
#4553=DIRECTION('',(1.,0.,0.));
#4554=DIRECTION('',(0.,0.,1.));
#4555=DIRECTION('center_axis',(0.,-1.,0.));
#4556=DIRECTION('ref_axis',(0.,0.,-1.));
#4557=DIRECTION('',(-1.,0.,0.));
#4558=DIRECTION('',(0.,0.,-1.));
#4559=DIRECTION('',(0.,0.,-1.));
#4560=DIRECTION('',(1.,0.,0.));
#4561=DIRECTION('',(0.,0.,-1.));
#4562=DIRECTION('center_axis',(0.,-1.,0.));
#4563=DIRECTION('ref_axis',(0.,0.,-1.));
#4564=DIRECTION('',(-1.,0.,0.));
#4565=DIRECTION('',(0.,0.,-1.));
#4566=DIRECTION('',(1.,0.,0.));
#4567=DIRECTION('',(0.,0.,1.));
#4568=DIRECTION('',(0.,0.,-1.));
#4569=DIRECTION('center_axis',(0.,-1.,0.));
#4570=DIRECTION('ref_axis',(0.,0.,-1.));
#4571=DIRECTION('center_axis',(0.,-1.,0.));
#4572=DIRECTION('ref_axis',(0.,0.,-1.));
#4573=DIRECTION('center_axis',(0.,-1.,0.));
#4574=DIRECTION('ref_axis',(0.,0.,-1.));
#4575=DIRECTION('center_axis',(1.,0.,1.85037170770859E-16));
#4576=DIRECTION('ref_axis',(1.85037170770859E-16,0.,-1.));
#4577=DIRECTION('',(0.,1.,0.));
#4578=DIRECTION('',(0.,1.,0.));
#4579=DIRECTION('',(2.39239978370404E-16,0.,-1.));
#4580=DIRECTION('',(0.,-1.,1.18423789293349E-15));
#4581=DIRECTION('',(-2.8421709430404E-16,2.8421709430404E-16,1.));
#4582=DIRECTION('center_axis',(0.,0.,1.));
#4583=DIRECTION('ref_axis',(1.,0.,0.));
#4584=DIRECTION('',(0.,-1.,0.));
#4585=DIRECTION('',(-1.,0.,0.));
#4586=DIRECTION('',(0.,1.,0.));
#4587=DIRECTION('',(0.,1.,0.));
#4588=DIRECTION('',(1.,0.,0.));
#4589=DIRECTION('',(0.,-1.,0.));
#4590=DIRECTION('',(-1.,0.,0.));
#4591=DIRECTION('',(0.,1.,0.));
#4592=DIRECTION('center_axis',(1.,0.,0.));
#4593=DIRECTION('ref_axis',(0.,0.,-1.));
#4594=DIRECTION('',(0.,1.,0.));
#4595=DIRECTION('',(0.,2.8421709430404E-16,1.));
#4596=DIRECTION('',(0.,-1.,0.));
#4597=DIRECTION('',(0.,0.,-1.));
#4598=DIRECTION('center_axis',(0.,-1.,0.));
#4599=DIRECTION('ref_axis',(0.,0.,-1.));
#4600=DIRECTION('center_axis',(0.,-1.,0.));
#4601=DIRECTION('ref_axis',(0.,0.,-1.));
#4602=DIRECTION('center_axis',(0.,-1.,0.));
#4603=DIRECTION('ref_axis',(0.,0.,-1.));
#4604=DIRECTION('center_axis',(1.,0.,0.));
#4605=DIRECTION('ref_axis',(0.,0.,-1.));
#4606=DIRECTION('',(0.,-1.,0.));
#4607=DIRECTION('',(0.,0.,-1.));
#4608=DIRECTION('',(0.,-1.,0.));
#4609=DIRECTION('',(0.,0.,-1.));
#4610=DIRECTION('',(0.,0.,1.));
#4611=DIRECTION('center_axis',(0.,1.,0.));
#4612=DIRECTION('ref_axis',(0.,0.,1.));
#4613=DIRECTION('center_axis',(0.,1.,0.));
#4614=DIRECTION('ref_axis',(0.,0.,1.));
#4615=DIRECTION('',(0.,0.,1.));
#4616=DIRECTION('center_axis',(-1.,0.,0.));
#4617=DIRECTION('ref_axis',(0.,0.,1.));
#4618=DIRECTION('',(0.,-1.,0.));
#4619=DIRECTION('center_axis',(-1.,0.,0.));
#4620=DIRECTION('ref_axis',(0.,0.,1.));
#4621=DIRECTION('',(0.,0.,1.));
#4622=DIRECTION('',(0.,-1.,0.));
#4623=DIRECTION('',(0.,0.,1.));
#4624=DIRECTION('',(0.,-1.,0.));
#4625=DIRECTION('center_axis',(1.,0.,0.));
#4626=DIRECTION('ref_axis',(0.,0.,-1.));
#4627=DIRECTION('center_axis',(1.,0.,0.));
#4628=DIRECTION('ref_axis',(0.,0.,-1.));
#4629=DIRECTION('',(0.,1.,0.));
#4630=DIRECTION('',(0.,0.,1.));
#4631=DIRECTION('',(0.,-1.,0.));
#4632=DIRECTION('',(0.,0.,-1.));
#4633=DIRECTION('',(0.,-1.,0.));
#4634=DIRECTION('',(0.,0.,-1.));
#4635=DIRECTION('center_axis',(0.,1.,0.));
#4636=DIRECTION('ref_axis',(0.,0.,1.));
#4637=DIRECTION('',(0.,0.,1.));
#4638=DIRECTION('center_axis',(0.,1.,0.));
#4639=DIRECTION('ref_axis',(0.,0.,1.));
#4640=DIRECTION('center_axis',(-1.,0.,0.));
#4641=DIRECTION('ref_axis',(0.,0.,1.));
#4642=DIRECTION('',(-3.86108475418265E-15,0.,1.));
#4643=DIRECTION('',(0.,-1.,0.));
#4644=DIRECTION('',(-3.86108475418265E-15,0.,1.));
#4645=DIRECTION('',(0.,-1.,0.));
#4646=DIRECTION('center_axis',(1.,0.,0.));
#4647=DIRECTION('ref_axis',(0.,0.,-1.));
#4648=DIRECTION('',(0.,0.,1.));
#4649=DIRECTION('',(0.,0.,-1.));
#4650=DIRECTION('',(0.,-1.,0.));
#4651=DIRECTION('',(0.,0.,-1.));
#4652=DIRECTION('',(0.,-1.,0.));
#4653=DIRECTION('center_axis',(0.,1.,0.));
#4654=DIRECTION('ref_axis',(0.,0.,1.));
#4655=DIRECTION('',(0.,0.,1.));
#4656=DIRECTION('center_axis',(0.,1.,0.));
#4657=DIRECTION('ref_axis',(0.,0.,1.));
#4658=DIRECTION('center_axis',(-1.,0.,0.));
#4659=DIRECTION('ref_axis',(0.,0.,1.));
#4660=DIRECTION('center_axis',(-1.,0.,0.));
#4661=DIRECTION('ref_axis',(0.,0.,1.));
#4662=DIRECTION('',(0.,-1.,0.));
#4663=DIRECTION('',(0.,-1.,0.));
#4664=DIRECTION('',(0.,0.,1.));
#4665=DIRECTION('',(0.,-1.,0.));
#4666=DIRECTION('',(0.,0.,1.));
#4667=DIRECTION('center_axis',(-1.,0.,0.));
#4668=DIRECTION('ref_axis',(0.,0.,1.));
#4669=DIRECTION('',(0.,-1.,0.));
#4670=DIRECTION('',(3.86108475418265E-15,0.,1.));
#4671=DIRECTION('',(0.,-1.,0.));
#4672=DIRECTION('',(3.86108475418265E-15,0.,1.));
#4673=DIRECTION('',(0.,0.,1.));
#4674=DIRECTION('center_axis',(1.,0.,0.));
#4675=DIRECTION('ref_axis',(0.,0.,-1.));
#4676=DIRECTION('',(0.,0.,1.));
#4677=DIRECTION('',(0.,1.,0.));
#4678=DIRECTION('center_axis',(1.,0.,0.));
#4679=DIRECTION('ref_axis',(0.,0.,-1.));
#4680=DIRECTION('',(0.,0.,-1.));
#4681=DIRECTION('',(0.,-1.,0.));
#4682=DIRECTION('',(0.,0.,-1.));
#4683=DIRECTION('',(0.,-1.,0.));
#4684=DIRECTION('center_axis',(0.,1.,0.));
#4685=DIRECTION('ref_axis',(0.,0.,1.));
#4686=DIRECTION('center_axis',(0.,1.,0.));
#4687=DIRECTION('ref_axis',(0.,0.,1.));
#4688=DIRECTION('center_axis',(0.,-1.,0.));
#4689=DIRECTION('ref_axis',(0.,0.,-1.));
#4690=DIRECTION('',(0.,0.,1.));
#4691=DIRECTION('',(0.,0.,1.));
#4692=DIRECTION('center_axis',(-1.,1.79068229778251E-16,0.));
#4693=DIRECTION('ref_axis',(0.,0.,1.));
#4694=DIRECTION('',(0.,0.,1.));
#4695=DIRECTION('center_axis',(0.,-1.,0.));
#4696=DIRECTION('ref_axis',(0.,0.,-1.));
#4697=DIRECTION('',(0.,0.,1.));
#4698=DIRECTION('center_axis',(-1.,-8.95341148891256E-17,0.));
#4699=DIRECTION('ref_axis',(0.,0.,1.));
#4700=DIRECTION('center_axis',(-1.,0.,0.));
#4701=DIRECTION('ref_axis',(0.,0.,1.));
#4702=DIRECTION('',(0.,0.,1.));
#4703=DIRECTION('',(0.,0.,1.));
#4704=DIRECTION('center_axis',(0.,1.,0.));
#4705=DIRECTION('ref_axis',(0.,0.,1.));
#4706=DIRECTION('',(0.,0.,1.));
#4707=DIRECTION('center_axis',(-1.,0.,0.));
#4708=DIRECTION('ref_axis',(0.,0.,1.));
#4709=DIRECTION('',(0.,0.,1.));
#4710=DIRECTION('center_axis',(0.,1.,0.));
#4711=DIRECTION('ref_axis',(0.,0.,1.));
#4712=DIRECTION('center_axis',(0.,0.,1.));
#4713=DIRECTION('ref_axis',(1.,0.,0.));
#4714=DIRECTION('',(0.,0.,1.));
#4715=DIRECTION('center_axis',(0.,0.,1.));
#4716=DIRECTION('ref_axis',(1.,0.,0.));
#4717=DIRECTION('',(0.,0.,1.));
#4718=DIRECTION('center_axis',(0.,0.,1.));
#4719=DIRECTION('ref_axis',(1.,0.,0.));
#4720=DIRECTION('',(0.,0.,1.));
#4721=DIRECTION('center_axis',(0.,0.,1.));
#4722=DIRECTION('ref_axis',(1.,0.,0.));
#4723=DIRECTION('',(0.,0.,1.));
#4724=DIRECTION('center_axis',(-1.85037170770859E-16,6.53551686595338E-16,
1.));
#4725=DIRECTION('ref_axis',(1.,0.,1.85037170770859E-16));
#4726=DIRECTION('',(-1.,0.,0.));
#4727=DIRECTION('',(0.,1.,0.));
#4728=DIRECTION('center_axis',(-1.85037170770859E-16,6.53551686595338E-16,
1.));
#4729=DIRECTION('ref_axis',(0.,-1.,6.53551686595338E-16));
#4730=DIRECTION('',(1.,0.,0.));
#4731=DIRECTION('',(0.,-1.,0.));
#4732=DIRECTION('',(1.,0.,0.));
#4733=DIRECTION('',(0.,-1.,0.));
#4734=DIRECTION('center_axis',(4.1086505480261E-32,1.,-2.22044604925031E-16));
#4735=DIRECTION('ref_axis',(0.,2.22044604925031E-16,1.));
#4736=DIRECTION('',(-1.,0.,0.));
#4737=DIRECTION('center_axis',(4.1086505480261E-32,1.,-2.22044604925031E-16));
#4738=DIRECTION('ref_axis',(0.,2.22044604925031E-16,1.));
#4739=DIRECTION('center_axis',(4.1086505480261E-32,1.,-2.22044604925031E-16));
#4740=DIRECTION('ref_axis',(0.,2.22044604925031E-16,1.));
#4741=DIRECTION('center_axis',(1.85037170770859E-16,8.71402248793784E-16,
-1.));
#4742=DIRECTION('ref_axis',(-1.,0.,-1.85037170770859E-16));
#4743=DIRECTION('center_axis',(1.85037170770859E-16,8.71402248793784E-16,
-1.));
#4744=DIRECTION('ref_axis',(0.,1.,8.71402248793784E-16));
#4745=DIRECTION('',(0.,-1.,-1.26882631385732E-15));
#4746=DIRECTION('',(0.,-1.,0.));
#4747=DIRECTION('',(-1.,0.,0.));
#4748=DIRECTION('',(0.,-1.,0.));
#4749=DIRECTION('',(-1.,0.,0.));
#4750=DIRECTION('center_axis',(1.85037170770859E-16,8.71402248793784E-16,
-1.));
#4751=DIRECTION('ref_axis',(-1.,0.,-1.85037170770859E-16));
#4752=DIRECTION('',(-1.,0.,0.));
#4753=DIRECTION('',(0.,1.,0.));
#4754=DIRECTION('center_axis',(1.85037170770859E-16,8.71402248793784E-16,
-1.));
#4755=DIRECTION('ref_axis',(0.,1.,8.71402248793784E-16));
#4756=DIRECTION('',(-1.,0.,0.));
#4757=DIRECTION('',(0.,-1.,0.));
#4758=DIRECTION('',(-1.,0.,0.));
#4759=DIRECTION('',(0.,-1.,0.));
#4760=DIRECTION('center_axis',(4.1086505480261E-32,1.,-2.22044604925031E-16));
#4761=DIRECTION('ref_axis',(0.,2.22044604925031E-16,1.));
#4762=DIRECTION('',(-1.,0.,0.));
#4763=DIRECTION('center_axis',(4.1086505480261E-32,1.,-2.22044604925031E-16));
#4764=DIRECTION('ref_axis',(0.,2.22044604925031E-16,1.));
#4765=DIRECTION('center_axis',(4.1086505480261E-32,1.,-2.22044604925031E-16));
#4766=DIRECTION('ref_axis',(0.,2.22044604925031E-16,1.));
#4767=DIRECTION('center_axis',(-1.85037170770859E-16,6.53551686595338E-16,
1.));
#4768=DIRECTION('ref_axis',(1.,0.,1.85037170770859E-16));
#4769=DIRECTION('center_axis',(-1.85037170770859E-16,6.53551686595338E-16,
1.));
#4770=DIRECTION('ref_axis',(0.,-1.,6.53551686595338E-16));
#4771=DIRECTION('',(0.,-1.,1.26882631385731E-15));
#4772=DIRECTION('',(0.,-1.,0.));
#4773=DIRECTION('',(1.,0.,1.28702825139422E-15));
#4774=DIRECTION('',(0.,-1.,0.));
#4775=DIRECTION('',(1.,0.,0.));
#4776=DIRECTION('center_axis',(0.,0.,1.));
#4777=DIRECTION('ref_axis',(1.,0.,0.));
#4778=DIRECTION('',(-1.,0.,0.));
#4779=DIRECTION('',(0.,-1.,0.));
#4780=DIRECTION('',(-1.,0.,0.));
#4781=DIRECTION('center_axis',(0.,0.,-1.));
#4782=DIRECTION('ref_axis',(-1.,0.,0.));
#4783=DIRECTION('',(0.,-1.,0.));
#4784=DIRECTION('',(1.,0.,0.));
#4785=DIRECTION('center_axis',(1.,0.,0.));
#4786=DIRECTION('ref_axis',(0.,0.,-1.));
#4787=DIRECTION('',(0.,0.,1.));
#4788=DIRECTION('center_axis',(-1.,0.,0.));
#4789=DIRECTION('ref_axis',(0.,0.,1.));
#4790=DIRECTION('',(0.,0.,-1.));
#4791=DIRECTION('',(0.,0.,-1.));
#4792=DIRECTION('center_axis',(0.,-1.,0.));
#4793=DIRECTION('ref_axis',(0.,0.,-1.));
#4794=DIRECTION('',(1.,0.,0.));
#4795=DIRECTION('',(0.,0.,-1.));
#4796=DIRECTION('',(-1.,0.,0.));
#4797=DIRECTION('',(0.,0.,1.));
#4798=DIRECTION('',(1.,0.,0.));
#4799=DIRECTION('',(0.,0.,1.));
#4800=DIRECTION('center_axis',(0.,-1.,0.));
#4801=DIRECTION('ref_axis',(0.,0.,-1.));
#4802=DIRECTION('center_axis',(0.,0.,1.));
#4803=DIRECTION('ref_axis',(1.,0.,0.));
#4804=DIRECTION('',(0.,-1.,0.));
#4805=DIRECTION('',(-1.,0.,0.));
#4806=DIRECTION('center_axis',(0.,0.,-1.));
#4807=DIRECTION('ref_axis',(-1.,0.,0.));
#4808=DIRECTION('',(0.,-1.,0.));
#4809=DIRECTION('',(1.,0.,0.));
#4810=DIRECTION('',(1.,0.,0.));
#4811=DIRECTION('center_axis',(-1.,0.,0.));
#4812=DIRECTION('ref_axis',(0.,0.,1.));
#4813=DIRECTION('',(0.,0.,-1.));
#4814=DIRECTION('',(0.,0.,-1.));
#4815=DIRECTION('center_axis',(1.,0.,0.));
#4816=DIRECTION('ref_axis',(0.,0.,-1.));
#4817=DIRECTION('',(0.,0.,1.));
#4818=DIRECTION('center_axis',(0.,1.,0.));
#4819=DIRECTION('ref_axis',(0.,0.,1.));
#4820=DIRECTION('',(-1.,0.,0.));
#4821=DIRECTION('',(0.,0.,1.));
#4822=DIRECTION('',(-1.,0.,0.));
#4823=DIRECTION('',(0.,0.,1.));
#4824=DIRECTION('',(1.,0.,0.));
#4825=DIRECTION('',(0.,0.,-1.));
#4826=DIRECTION('center_axis',(0.,1.,0.));
#4827=DIRECTION('ref_axis',(0.,0.,1.));
#4828=DIRECTION('center_axis',(-1.,0.,0.));
#4829=DIRECTION('ref_axis',(0.,0.,1.));
#4830=DIRECTION('',(0.,-1.,0.));
#4831=DIRECTION('',(0.,0.,-1.));
#4832=DIRECTION('center_axis',(1.,0.,0.));
#4833=DIRECTION('ref_axis',(0.,0.,-1.));
#4834=DIRECTION('',(0.,-1.,0.));
#4835=DIRECTION('',(0.,0.,1.));
#4836=DIRECTION('',(0.,0.,1.));
#4837=DIRECTION('center_axis',(0.,0.,-1.));
#4838=DIRECTION('ref_axis',(-1.,0.,0.));
#4839=DIRECTION('',(1.,0.,0.));
#4840=DIRECTION('',(1.,0.,0.));
#4841=DIRECTION('center_axis',(0.,0.,1.));
#4842=DIRECTION('ref_axis',(1.,0.,0.));
#4843=DIRECTION('',(-1.,0.,0.));
#4844=DIRECTION('center_axis',(0.,-1.,0.));
#4845=DIRECTION('ref_axis',(0.,0.,-1.));
#4846=DIRECTION('',(0.,0.,-1.));
#4847=DIRECTION('',(-1.,0.,0.));
#4848=DIRECTION('',(0.,0.,-1.));
#4849=DIRECTION('',(-1.,0.,0.));
#4850=DIRECTION('',(0.,0.,1.));
#4851=DIRECTION('',(1.,0.,0.));
#4852=DIRECTION('center_axis',(0.,-1.,0.));
#4853=DIRECTION('ref_axis',(0.,0.,-1.));
#4854=DIRECTION('center_axis',(0.,0.,-1.));
#4855=DIRECTION('ref_axis',(-1.,0.,0.));
#4856=DIRECTION('',(0.,-1.,0.));
#4857=DIRECTION('',(1.,0.,0.));
#4858=DIRECTION('center_axis',(0.,0.,1.));
#4859=DIRECTION('ref_axis',(1.,0.,0.));
#4860=DIRECTION('',(0.,-1.,0.));
#4861=DIRECTION('',(-1.,0.,0.));
#4862=DIRECTION('',(-1.,0.,0.));
#4863=DIRECTION('center_axis',(1.,0.,0.));
#4864=DIRECTION('ref_axis',(0.,0.,-1.));
#4865=DIRECTION('',(0.,0.,1.));
#4866=DIRECTION('',(0.,0.,1.));
#4867=DIRECTION('center_axis',(-1.,0.,0.));
#4868=DIRECTION('ref_axis',(0.,0.,1.));
#4869=DIRECTION('',(0.,0.,-1.));
#4870=DIRECTION('center_axis',(0.,1.,0.));
#4871=DIRECTION('ref_axis',(0.,0.,1.));
#4872=DIRECTION('',(1.,0.,0.));
#4873=DIRECTION('',(0.,0.,-1.));
#4874=DIRECTION('',(1.,0.,0.));
#4875=DIRECTION('',(0.,0.,-1.));
#4876=DIRECTION('',(-1.,0.,0.));
#4877=DIRECTION('',(0.,0.,1.));
#4878=DIRECTION('center_axis',(0.,1.,0.));
#4879=DIRECTION('ref_axis',(0.,0.,1.));
#4880=DIRECTION('center_axis',(0.,0.,1.));
#4881=DIRECTION('ref_axis',(1.,0.,0.));
#4882=DIRECTION('',(-1.,0.,0.));
#4883=DIRECTION('center_axis',(0.,0.,-1.));
#4884=DIRECTION('ref_axis',(-1.,0.,0.));
#4885=DIRECTION('',(1.,0.,0.));
#4886=DIRECTION('',(1.,0.,0.));
#4887=DIRECTION('center_axis',(0.,-1.,0.));
#4888=DIRECTION('ref_axis',(0.,0.,-1.));
#4889=DIRECTION('center_axis',(0.,-1.,0.));
#4890=DIRECTION('ref_axis',(0.,0.,-1.));
#4891=DIRECTION('center_axis',(0.,0.,1.));
#4892=DIRECTION('ref_axis',(1.,0.,0.));
#4893=DIRECTION('',(-1.,0.,0.));
#4894=DIRECTION('',(-1.,0.,0.));
#4895=DIRECTION('center_axis',(0.,0.,-1.));
#4896=DIRECTION('ref_axis',(-1.,0.,0.));
#4897=DIRECTION('',(1.,0.,0.));
#4898=DIRECTION('center_axis',(0.,1.,0.));
#4899=DIRECTION('ref_axis',(0.,0.,1.));
#4900=DIRECTION('center_axis',(0.,1.,0.));
#4901=DIRECTION('ref_axis',(0.,0.,1.));
#4902=DIRECTION('center_axis',(0.,0.,-1.));
#4903=DIRECTION('ref_axis',(-1.,0.,0.));
#4904=DIRECTION('center_axis',(0.,0.,1.));
#4905=DIRECTION('ref_axis',(1.,0.,0.));
#4906=DIRECTION('center_axis',(-0.707106781186548,0.,-0.707106781186548));
#4907=DIRECTION('ref_axis',(0.707106781186548,0.,-0.707106781186548));
#4908=DIRECTION('center_axis',(0.,-1.,0.));
#4909=DIRECTION('ref_axis',(0.,0.,-1.));
#4910=DIRECTION('center_axis',(0.,-1.,0.));
#4911=DIRECTION('ref_axis',(0.,0.,-1.));
#4912=DIRECTION('center_axis',(1.,0.,0.));
#4913=DIRECTION('ref_axis',(0.,0.,-1.));
#4914=DIRECTION('center_axis',(0.707106781186548,0.,-0.707106781186548));
#4915=DIRECTION('ref_axis',(0.707106781186548,0.,0.707106781186548));
#4916=DIRECTION('center_axis',(-1.,0.,0.));
#4917=DIRECTION('ref_axis',(0.,0.,1.));
#4918=DIRECTION('center_axis',(-1.,0.,0.));
#4919=DIRECTION('ref_axis',(0.,0.,1.));
#4920=DIRECTION('center_axis',(0.,0.,-1.));
#4921=DIRECTION('ref_axis',(-1.,0.,0.));
#4922=DIRECTION('center_axis',(-0.707106781186547,0.,-0.707106781186548));
#4923=DIRECTION('ref_axis',(0.707106781186548,0.,-0.707106781186547));
#4924=DIRECTION('center_axis',(-1.,0.,0.));
#4925=DIRECTION('ref_axis',(0.,0.,1.));
#4926=DIRECTION('center_axis',(-0.707106781186548,0.,0.707106781186547));
#4927=DIRECTION('ref_axis',(-0.707106781186547,0.,-0.707106781186548));
#4928=DIRECTION('center_axis',(1.,0.,1.85037170770859E-16));
#4929=DIRECTION('ref_axis',(1.85037170770859E-16,0.,-1.));
#4930=DIRECTION('center_axis',(1.,0.,0.));
#4931=DIRECTION('ref_axis',(0.,0.,-1.));
#4932=DIRECTION('center_axis',(-1.85037170770859E-16,0.,1.));
#4933=DIRECTION('ref_axis',(1.,0.,1.85037170770859E-16));
#4934=DIRECTION('center_axis',(1.85037170770859E-16,8.71402248793784E-16,
-1.));
#4935=DIRECTION('ref_axis',(0.,1.,8.71402248793784E-16));
#4936=DIRECTION('center_axis',(1.85037170770859E-16,8.71402248793784E-16,
-1.));
#4937=DIRECTION('ref_axis',(-1.,0.,0.));
#4938=DIRECTION('center_axis',(0.,-1.,0.));
#4939=DIRECTION('ref_axis',(0.,0.,-1.));
#4940=DIRECTION('center_axis',(-1.61241806720166E-31,1.,8.71402248793784E-16));
#4941=DIRECTION('ref_axis',(0.,-8.71402248793784E-16,1.));
#4942=DIRECTION('center_axis',(-1.,0.,-1.85037170770859E-16));
#4943=DIRECTION('ref_axis',(-1.85037170770859E-16,0.,1.));
#4944=DIRECTION('center_axis',(-1.,0.,0.));
#4945=DIRECTION('ref_axis',(0.,0.,1.));
#4946=DIRECTION('center_axis',(-0.707106781186548,0.,0.707106781186547));
#4947=DIRECTION('ref_axis',(-0.707106781186547,0.,-0.707106781186548));
#4948=DIRECTION('center_axis',(0.,1.,8.71402248793784E-16));
#4949=DIRECTION('ref_axis',(0.,-8.71402248793784E-16,1.));
#4950=DIRECTION('center_axis',(0.,-1.,0.));
#4951=DIRECTION('ref_axis',(0.,0.,-1.));
#4952=DIRECTION('center_axis',(0.,0.,-1.));
#4953=DIRECTION('ref_axis',(-1.,0.,0.));
#4954=DIRECTION('center_axis',(-0.707106781186548,0.,-0.707106781186548));
#4955=DIRECTION('ref_axis',(0.707106781186548,0.,-0.707106781186548));
#4956=DIRECTION('center_axis',(1.85037170770859E-16,8.71402248793784E-16,
-1.));
#4957=DIRECTION('ref_axis',(-1.,0.,0.));
#4958=DIRECTION('center_axis',(1.85037170770859E-16,8.71402248793784E-16,
-1.));
#4959=DIRECTION('ref_axis',(0.,1.,8.71402248793784E-16));
#4960=DIRECTION('center_axis',(-1.,0.,0.));
#4961=DIRECTION('ref_axis',(0.,0.,1.));
#4962=DIRECTION('center_axis',(-0.707106781186548,0.,0.707106781186548));
#4963=DIRECTION('ref_axis',(-0.707106781186548,0.,-0.707106781186548));
#4964=DIRECTION('center_axis',(0.,0.,-1.));
#4965=DIRECTION('ref_axis',(-1.,0.,0.));
#4966=DIRECTION('center_axis',(-0.707106781186548,0.,-0.707106781186548));
#4967=DIRECTION('ref_axis',(0.707106781186548,0.,-0.707106781186548));
#4968=DIRECTION('center_axis',(0.,0.,-1.));
#4969=DIRECTION('ref_axis',(-1.,0.,0.));
#4970=DIRECTION('center_axis',(0.,0.,1.));
#4971=DIRECTION('ref_axis',(1.,0.,0.));
#4972=DIRECTION('center_axis',(1.,0.,0.));
#4973=DIRECTION('ref_axis',(0.,0.,-1.));
#4974=DIRECTION('center_axis',(1.,0.,0.));
#4975=DIRECTION('ref_axis',(0.,0.,-1.));
#4976=DIRECTION('center_axis',(1.,0.,0.));
#4977=DIRECTION('ref_axis',(0.,0.,-1.));
#4978=DIRECTION('center_axis',(0.,-1.,0.));
#4979=DIRECTION('ref_axis',(0.,0.,-1.));
#4980=DIRECTION('center_axis',(0.,1.,0.));
#4981=DIRECTION('ref_axis',(0.,0.,1.));
#4982=DIRECTION('center_axis',(0.,0.,1.));
#4983=DIRECTION('ref_axis',(1.,0.,0.));
#4984=DIRECTION('center_axis',(0.,0.,-1.));
#4985=DIRECTION('ref_axis',(-1.,0.,0.));
#4986=DIRECTION('center_axis',(0.707106781186548,0.,0.707106781186548));
#4987=DIRECTION('ref_axis',(-0.707106781186548,0.,0.707106781186548));
#4988=DIRECTION('center_axis',(0.,-1.,0.));
#4989=DIRECTION('ref_axis',(0.,0.,-1.));
#4990=DIRECTION('center_axis',(0.,-1.,0.));
#4991=DIRECTION('ref_axis',(0.,0.,-1.));
#4992=DIRECTION('center_axis',(-1.,0.,0.));
#4993=DIRECTION('ref_axis',(0.,0.,1.));
#4994=DIRECTION('center_axis',(-0.707106781186548,0.,0.707106781186548));
#4995=DIRECTION('ref_axis',(-0.707106781186548,0.,-0.707106781186548));
#4996=DIRECTION('center_axis',(1.,0.,0.));
#4997=DIRECTION('ref_axis',(0.,0.,-1.));
#4998=DIRECTION('center_axis',(1.,0.,0.));
#4999=DIRECTION('ref_axis',(0.,0.,-1.));
#5000=DIRECTION('center_axis',(0.,0.,1.));
#5001=DIRECTION('ref_axis',(1.,0.,0.));
#5002=DIRECTION('center_axis',(0.707106781186547,0.,0.707106781186548));
#5003=DIRECTION('ref_axis',(-0.707106781186548,0.,0.707106781186547));
#5004=DIRECTION('center_axis',(-1.,0.,0.));
#5005=DIRECTION('ref_axis',(0.,0.,1.));
#5006=DIRECTION('center_axis',(-0.707106781186548,0.,0.707106781186548));
#5007=DIRECTION('ref_axis',(-0.707106781186548,0.,-0.707106781186548));
#5008=DIRECTION('center_axis',(-1.,0.,-1.85037170770859E-16));
#5009=DIRECTION('ref_axis',(-1.85037170770859E-16,0.,1.));
#5010=DIRECTION('center_axis',(-1.,0.,0.));
#5011=DIRECTION('ref_axis',(0.,0.,1.));
#5012=DIRECTION('center_axis',(0.,0.,1.));
#5013=DIRECTION('ref_axis',(1.,0.,0.));
#5014=DIRECTION('center_axis',(-1.85037170770859E-16,6.53551686595338E-16,
1.));
#5015=DIRECTION('ref_axis',(0.,-1.,6.53551686595338E-16));
#5016=DIRECTION('center_axis',(-1.85037170770859E-16,6.53551686595338E-16,
1.));
#5017=DIRECTION('ref_axis',(1.,0.,0.));
#5018=DIRECTION('center_axis',(0.,-1.,0.));
#5019=DIRECTION('ref_axis',(0.,0.,-1.));
#5020=DIRECTION('center_axis',(0.,-1.,6.53551686595338E-16));
#5021=DIRECTION('ref_axis',(0.,-6.53551686595338E-16,-1.));
#5022=DIRECTION('center_axis',(0.,1.,0.));
#5023=DIRECTION('ref_axis',(0.,0.,1.));
#5024=DIRECTION('center_axis',(0.,-1.,0.));
#5025=DIRECTION('ref_axis',(0.,0.,-1.));
#5026=DIRECTION('center_axis',(0.,0.,1.));
#5027=DIRECTION('ref_axis',(1.,0.,0.));
#5028=DIRECTION('center_axis',(0.707106781186548,0.,-0.707106781186548));
#5029=DIRECTION('ref_axis',(0.707106781186548,0.,0.707106781186548));
#5030=DIRECTION('center_axis',(0.,0.,-1.));
#5031=DIRECTION('ref_axis',(-1.,0.,0.));
#5032=DIRECTION('center_axis',(-1.,0.,0.));
#5033=DIRECTION('ref_axis',(0.,0.,1.));
#5034=DIRECTION('center_axis',(-1.,0.,0.));
#5035=DIRECTION('ref_axis',(0.,0.,1.));
#5036=DIRECTION('center_axis',(1.,0.,0.));
#5037=DIRECTION('ref_axis',(0.,0.,-1.));
#5038=DIRECTION('center_axis',(0.707106781186548,0.,0.707106781186548));
#5039=DIRECTION('ref_axis',(0.707106781186548,0.,-0.707106781186548));
#5040=DIRECTION('center_axis',(1.,0.,0.));
#5041=DIRECTION('ref_axis',(0.,0.,-1.));
#5042=DIRECTION('center_axis',(0.707106781186547,0.,0.707106781186548));
#5043=DIRECTION('ref_axis',(0.707106781186548,0.,-0.707106781186547));
#5044=DIRECTION('center_axis',(0.,0.,1.));
#5045=DIRECTION('ref_axis',(1.,0.,0.));
#5046=DIRECTION('center_axis',(0.707106781186548,0.,-0.707106781186547));
#5047=DIRECTION('ref_axis',(0.707106781186547,0.,0.707106781186548));
#5048=DIRECTION('center_axis',(1.85037170770859E-16,0.,-1.));
#5049=DIRECTION('ref_axis',(-1.,0.,-1.85037170770859E-16));
#5050=DIRECTION('center_axis',(-1.85037170770859E-16,6.53551686595338E-16,
1.));
#5051=DIRECTION('ref_axis',(0.,-1.,6.53551686595338E-16));
#5052=DIRECTION('center_axis',(1.,0.,1.85037170770859E-16));
#5053=DIRECTION('ref_axis',(1.85037170770859E-16,0.,-1.));
#5054=DIRECTION('center_axis',(1.,0.,0.));
#5055=DIRECTION('ref_axis',(0.,0.,-1.));
#5056=DIRECTION('center_axis',(-1.85037170770859E-16,6.53551686595338E-16,
1.));
#5057=DIRECTION('ref_axis',(1.,0.,0.));
#5058=DIRECTION('center_axis',(0.,-1.,0.));
#5059=DIRECTION('ref_axis',(0.,0.,-1.));
#5060=DIRECTION('center_axis',(-1.20931355040125E-31,-1.,6.53551686595338E-16));
#5061=DIRECTION('ref_axis',(0.,-6.53551686595338E-16,-1.));
#5062=DIRECTION('center_axis',(0.,-1.,0.));
#5063=DIRECTION('ref_axis',(0.,0.,-1.));
#5064=DIRECTION('',(0.,-1.,0.));
#5065=DIRECTION('center_axis',(0.,-1.,0.));
#5066=DIRECTION('ref_axis',(0.,0.,-1.));
#5067=DIRECTION('',(0.,-1.,0.));
#5608=CARTESIAN_POINT('',(0.,0.,0.));
#5609=CARTESIAN_POINT('Origin',(-800.,-535.,300.));
#5610=CARTESIAN_POINT('',(176.,-505.,300.));
#5611=CARTESIAN_POINT('',(-195.,-505.,300.));
#5612=CARTESIAN_POINT('',(176.,-505.,300.));
#5613=CARTESIAN_POINT('',(176.,-533.,300.));
#5614=CARTESIAN_POINT('',(176.,-533.,300.));
#5615=CARTESIAN_POINT('',(250.,-533.,300.));
#5616=CARTESIAN_POINT('',(176.,-533.,300.));
#5617=CARTESIAN_POINT('',(250.,-285.,300.));
#5618=CARTESIAN_POINT('',(250.,-533.,300.));
#5619=CARTESIAN_POINT('',(-800.,-285.,300.));
#5620=CARTESIAN_POINT('',(-800.,-285.,300.));
#5621=CARTESIAN_POINT('',(-800.,-533.,300.));
#5622=CARTESIAN_POINT('',(-800.,-533.,300.));
#5623=CARTESIAN_POINT('',(-726.,-533.,300.));
#5624=CARTESIAN_POINT('',(-800.,-533.,300.));
#5625=CARTESIAN_POINT('',(-726.,-505.,300.));
#5626=CARTESIAN_POINT('',(-726.,-505.,300.));
#5627=CARTESIAN_POINT('',(-355.,-505.,300.));
#5628=CARTESIAN_POINT('',(-355.,-505.,300.));
#5629=CARTESIAN_POINT('',(-355.,-534.,300.));
#5630=CARTESIAN_POINT('',(-355.,-534.,300.));
#5631=CARTESIAN_POINT('',(-195.,-534.,300.));
#5632=CARTESIAN_POINT('',(-355.,-534.,300.));
#5633=CARTESIAN_POINT('',(-195.,-505.,300.));
#5634=CARTESIAN_POINT('',(208.,-325.693069306929,300.));
#5635=CARTESIAN_POINT('Origin',(210.,-325.693069306929,300.));
#5636=CARTESIAN_POINT('',(-122.,-325.693069306929,300.));
#5637=CARTESIAN_POINT('Origin',(-120.,-325.693069306929,300.));
#5638=CARTESIAN_POINT('',(208.,-490.693069306929,300.));
#5639=CARTESIAN_POINT('Origin',(210.,-490.693069306929,300.));
#5640=CARTESIAN_POINT('',(-122.,-490.693069306929,300.));
#5641=CARTESIAN_POINT('Origin',(-120.,-490.693069306929,300.));
#5642=CARTESIAN_POINT('',(-115.,-330.693069306929,300.));
#5643=CARTESIAN_POINT('',(-115.,-485.693069306929,300.));
#5644=CARTESIAN_POINT('',(-115.,-330.693069306929,300.));
#5645=CARTESIAN_POINT('',(205.,-330.693069306929,300.));
#5646=CARTESIAN_POINT('',(-115.,-330.693069306929,300.));
#5647=CARTESIAN_POINT('',(205.,-485.693069306929,300.));
#5648=CARTESIAN_POINT('',(205.,-330.693069306929,300.));
#5649=CARTESIAN_POINT('',(-115.,-485.693069306929,300.));
#5650=CARTESIAN_POINT('',(-435.,-330.693069306929,300.));
#5651=CARTESIAN_POINT('',(-755.,-330.693069306929,300.));
#5652=CARTESIAN_POINT('',(-435.,-330.693069306929,300.));
#5653=CARTESIAN_POINT('',(-435.,-485.693069306929,300.));
#5654=CARTESIAN_POINT('',(-435.,-330.693069306929,300.));
#5655=CARTESIAN_POINT('',(-755.,-485.693069306929,300.));
#5656=CARTESIAN_POINT('',(-435.,-485.693069306929,300.));
#5657=CARTESIAN_POINT('',(-755.,-330.693069306929,300.));
#5658=CARTESIAN_POINT('Origin',(-800.,-535.,300.));
#5659=CARTESIAN_POINT('',(-800.,-533.,-251.));
#5660=CARTESIAN_POINT('',(-800.,-505.,-251.));
#5661=CARTESIAN_POINT('',(-800.,-533.,-251.));
#5662=CARTESIAN_POINT('',(-800.,-505.,251.));
#5663=CARTESIAN_POINT('',(-800.,-505.,-251.));
#5664=CARTESIAN_POINT('',(-800.,-533.,251.));
#5665=CARTESIAN_POINT('',(-800.,-505.,251.));
#5666=CARTESIAN_POINT('',(-800.,-533.,251.));
#5667=CARTESIAN_POINT('',(-800.,-285.,-300.));
#5668=CARTESIAN_POINT('',(-800.,-285.,300.));
#5669=CARTESIAN_POINT('',(-800.,-533.,-300.));
#5670=CARTESIAN_POINT('',(-800.,-533.,-300.));
#5671=CARTESIAN_POINT('',(-800.,-533.,-300.));
#5672=CARTESIAN_POINT('Origin',(-800.,-535.,-300.));
#5673=CARTESIAN_POINT('',(-355.,-505.,-300.));
#5674=CARTESIAN_POINT('',(-726.,-505.,-300.));
#5675=CARTESIAN_POINT('',(-355.,-505.,-300.));
#5676=CARTESIAN_POINT('',(-726.,-533.,-300.));
#5677=CARTESIAN_POINT('',(-726.,-505.,-300.));
#5678=CARTESIAN_POINT('',(-726.,-533.,-300.));
#5679=CARTESIAN_POINT('',(250.,-285.,-300.));
#5680=CARTESIAN_POINT('',(-800.,-285.,-300.));
#5681=CARTESIAN_POINT('',(250.,-533.,-300.));
#5682=CARTESIAN_POINT('',(250.,-533.,-300.));
#5683=CARTESIAN_POINT('',(176.,-533.,-300.));
#5684=CARTESIAN_POINT('',(250.,-533.,-300.));
#5685=CARTESIAN_POINT('',(176.,-505.,-300.));
#5686=CARTESIAN_POINT('',(176.,-533.,-300.));
#5687=CARTESIAN_POINT('',(-195.,-505.,-300.));
#5688=CARTESIAN_POINT('',(176.,-505.,-300.));
#5689=CARTESIAN_POINT('',(-195.,-534.,-300.));
#5690=CARTESIAN_POINT('',(-195.,-505.,-300.));
#5691=CARTESIAN_POINT('',(-355.,-534.,-300.));
#5692=CARTESIAN_POINT('',(-195.,-534.,-300.));
#5693=CARTESIAN_POINT('',(-355.,-534.,-300.));
#5694=CARTESIAN_POINT('Origin',(250.,-535.,300.));
#5695=CARTESIAN_POINT('',(250.,-505.,251.));
#5696=CARTESIAN_POINT('',(250.,-505.,-251.));
#5697=CARTESIAN_POINT('',(250.,-505.,251.));
#5698=CARTESIAN_POINT('',(250.,-533.,-251.));
#5699=CARTESIAN_POINT('',(250.,-505.,-251.));
#5700=CARTESIAN_POINT('',(250.,-533.,-251.));
#5701=CARTESIAN_POINT('',(250.,-285.,300.));
#5702=CARTESIAN_POINT('',(250.,-533.,251.));
#5703=CARTESIAN_POINT('',(250.,-533.,300.));
#5704=CARTESIAN_POINT('',(250.,-533.,251.));
#5705=CARTESIAN_POINT('Origin',(0.,-535.,0.));
#5706=CARTESIAN_POINT('',(-800.,-535.,-250.));
#5707=CARTESIAN_POINT('',(-797.,-535.,-250.));
#5708=CARTESIAN_POINT('',(-800.,-535.,-250.));
#5709=CARTESIAN_POINT('',(-800.,-535.,-300.));
#5710=CARTESIAN_POINT('',(-800.,-535.,-250.));
#5711=CARTESIAN_POINT('',(-725.,-535.,-300.));
#5712=CARTESIAN_POINT('',(-800.,-535.,-300.));
#5713=CARTESIAN_POINT('',(-725.,-535.,-297.));
#5714=CARTESIAN_POINT('',(-725.,-535.,-297.));
#5715=CARTESIAN_POINT('',(-797.,-535.,-297.));
#5716=CARTESIAN_POINT('',(-797.,-535.,-297.));
#5717=CARTESIAN_POINT('',(-797.,-535.,-250.));
#5718=CARTESIAN_POINT('Origin',(0.,-535.,0.));
#5719=CARTESIAN_POINT('',(247.,-535.,-250.));
#5720=CARTESIAN_POINT('',(250.,-535.,-250.));
#5721=CARTESIAN_POINT('',(247.,-535.,-250.));
#5722=CARTESIAN_POINT('',(247.,-535.,-297.));
#5723=CARTESIAN_POINT('',(247.,-535.,-250.));
#5724=CARTESIAN_POINT('',(175.,-535.,-297.));
#5725=CARTESIAN_POINT('',(175.,-535.,-297.));
#5726=CARTESIAN_POINT('',(175.,-535.,-300.));
#5727=CARTESIAN_POINT('',(175.,-535.,-300.));
#5728=CARTESIAN_POINT('',(250.,-535.,-300.));
#5729=CARTESIAN_POINT('',(175.,-535.,-300.));
#5730=CARTESIAN_POINT('',(250.,-535.,-250.));
#5731=CARTESIAN_POINT('Origin',(-800.,-535.,297.));
#5732=CARTESIAN_POINT('',(175.,-505.,297.));
#5733=CARTESIAN_POINT('',(-195.,-505.,297.));
#5734=CARTESIAN_POINT('',(175.,-505.,297.));
#5735=CARTESIAN_POINT('',(-195.,-535.,297.));
#5736=CARTESIAN_POINT('',(-195.,-505.,297.));
#5737=CARTESIAN_POINT('',(-355.,-535.,297.));
#5738=CARTESIAN_POINT('',(-355.,-535.,297.));
#5739=CARTESIAN_POINT('',(-355.,-505.,297.));
#5740=CARTESIAN_POINT('',(-355.,-535.,297.));
#5741=CARTESIAN_POINT('',(-725.,-505.,297.));
#5742=CARTESIAN_POINT('',(-355.,-505.,297.));
#5743=CARTESIAN_POINT('',(-725.,-535.,297.));
#5744=CARTESIAN_POINT('',(-725.,-505.,297.));
#5745=CARTESIAN_POINT('',(-797.,-535.,297.));
#5746=CARTESIAN_POINT('',(-797.,-535.,297.));
#5747=CARTESIAN_POINT('',(-797.,-288.,297.));
#5748=CARTESIAN_POINT('',(-797.,-535.,297.));
#5749=CARTESIAN_POINT('',(247.,-288.,297.));
#5750=CARTESIAN_POINT('',(-797.,-288.,297.));
#5751=CARTESIAN_POINT('',(247.,-535.,297.));
#5752=CARTESIAN_POINT('',(247.,-535.,297.));
#5753=CARTESIAN_POINT('',(175.,-535.,297.));
#5754=CARTESIAN_POINT('',(175.,-535.,297.));
#5755=CARTESIAN_POINT('',(175.,-535.,297.));
#5756=CARTESIAN_POINT('',(-435.,-330.693069306929,297.));
#5757=CARTESIAN_POINT('',(-435.,-485.693069306929,297.));
#5758=CARTESIAN_POINT('',(-435.,-330.693069306929,297.));
#5759=CARTESIAN_POINT('',(-755.,-330.693069306929,297.));
#5760=CARTESIAN_POINT('',(-435.,-330.693069306929,297.));
#5761=CARTESIAN_POINT('',(-755.,-485.693069306929,297.));
#5762=CARTESIAN_POINT('',(-755.,-330.693069306929,297.));
#5763=CARTESIAN_POINT('',(-435.,-485.693069306929,297.));
#5764=CARTESIAN_POINT('',(208.,-325.693069306929,297.));
#5765=CARTESIAN_POINT('Origin',(210.,-325.693069306929,297.));
#5766=CARTESIAN_POINT('',(-122.,-325.693069306929,297.));
#5767=CARTESIAN_POINT('Origin',(-120.,-325.693069306929,297.));
#5768=CARTESIAN_POINT('',(208.,-490.693069306929,297.));
#5769=CARTESIAN_POINT('Origin',(210.,-490.693069306929,297.));
#5770=CARTESIAN_POINT('',(-122.,-490.693069306929,297.));
#5771=CARTESIAN_POINT('Origin',(-120.,-490.693069306929,297.));
#5772=CARTESIAN_POINT('',(-115.,-330.693069306929,297.));
#5773=CARTESIAN_POINT('',(205.,-330.693069306929,297.));
#5774=CARTESIAN_POINT('',(-115.,-330.693069306929,297.));
#5775=CARTESIAN_POINT('',(-115.,-485.693069306929,297.));
#5776=CARTESIAN_POINT('',(-115.,-330.693069306929,297.));
#5777=CARTESIAN_POINT('',(205.,-485.693069306929,297.));
#5778=CARTESIAN_POINT('',(-115.,-485.693069306929,297.));
#5779=CARTESIAN_POINT('',(205.,-330.693069306929,297.));
#5780=CARTESIAN_POINT('Origin',(0.,-535.,0.));
#5781=CARTESIAN_POINT('',(-195.,-535.,-297.));
#5782=CARTESIAN_POINT('',(-195.,-535.,-300.));
#5783=CARTESIAN_POINT('',(-195.,-535.,-297.));
#5784=CARTESIAN_POINT('',(-355.,-535.,-297.));
#5785=CARTESIAN_POINT('',(-355.,-535.,-297.));
#5786=CARTESIAN_POINT('',(-355.,-535.,-300.));
#5787=CARTESIAN_POINT('',(-355.,-535.,-300.));
#5788=CARTESIAN_POINT('',(-355.,-535.,-300.));
#5789=CARTESIAN_POINT('Origin',(0.,-535.,0.));
#5790=CARTESIAN_POINT('',(-195.,-535.,300.));
#5791=CARTESIAN_POINT('',(-195.,-535.,300.));
#5792=CARTESIAN_POINT('',(-355.,-535.,300.));
#5793=CARTESIAN_POINT('',(-355.,-535.,300.));
#5794=CARTESIAN_POINT('',(-355.,-535.,297.));
#5795=CARTESIAN_POINT('Origin',(0.,-535.,0.));
#5796=CARTESIAN_POINT('',(-797.,-535.,250.));
#5797=CARTESIAN_POINT('',(-800.,-535.,250.));
#5798=CARTESIAN_POINT('',(-797.,-535.,250.));
#5799=CARTESIAN_POINT('',(-797.,-535.,297.));
#5800=CARTESIAN_POINT('',(-725.,-535.,300.));
#5801=CARTESIAN_POINT('',(-725.,-535.,300.));
#5802=CARTESIAN_POINT('',(-800.,-535.,300.));
#5803=CARTESIAN_POINT('',(-800.,-535.,300.));
#5804=CARTESIAN_POINT('',(-800.,-535.,300.));
#5805=CARTESIAN_POINT('Origin',(0.,-535.,0.));
#5806=CARTESIAN_POINT('',(250.,-535.,250.));
#5807=CARTESIAN_POINT('',(247.,-535.,250.));
#5808=CARTESIAN_POINT('',(250.,-535.,250.));
#5809=CARTESIAN_POINT('',(250.,-535.,300.));
#5810=CARTESIAN_POINT('',(250.,-535.,300.));
#5811=CARTESIAN_POINT('',(175.,-535.,300.));
#5812=CARTESIAN_POINT('',(175.,-535.,300.));
#5813=CARTESIAN_POINT('',(175.,-535.,297.));
#5814=CARTESIAN_POINT('',(247.,-535.,297.));
#5815=CARTESIAN_POINT('Origin',(0.,-285.,0.));
#5816=CARTESIAN_POINT('',(-500.,-285.,35.));
#5817=CARTESIAN_POINT('Origin',(-500.,-285.,-6.12323399573677E-14));
#5818=CARTESIAN_POINT('',(-4.28626379701574E-15,-285.,35.));
#5819=CARTESIAN_POINT('Origin',(0.,-285.,0.));
#5820=CARTESIAN_POINT('Origin',(-797.,-535.,300.));
#5821=CARTESIAN_POINT('',(-797.,-505.,-250.));
#5822=CARTESIAN_POINT('',(-797.,-535.,-250.));
#5823=CARTESIAN_POINT('',(-797.,-288.,-297.));
#5824=CARTESIAN_POINT('',(-797.,-535.,-297.));
#5825=CARTESIAN_POINT('',(-797.,-288.,297.));
#5826=CARTESIAN_POINT('',(-797.,-505.,250.));
#5827=CARTESIAN_POINT('',(-797.,-505.,250.));
#5828=CARTESIAN_POINT('',(-797.,-505.,-250.));
#5829=CARTESIAN_POINT('Origin',(-800.,-535.,-297.));
#5830=CARTESIAN_POINT('',(-195.,-505.,-297.));
#5831=CARTESIAN_POINT('',(-195.,-505.,-297.));
#5832=CARTESIAN_POINT('',(175.,-505.,-297.));
#5833=CARTESIAN_POINT('',(175.,-505.,-297.));
#5834=CARTESIAN_POINT('',(175.,-535.,-297.));
#5835=CARTESIAN_POINT('',(247.,-288.,-297.));
#5836=CARTESIAN_POINT('',(247.,-535.,-297.));
#5837=CARTESIAN_POINT('',(-797.,-288.,-297.));
#5838=CARTESIAN_POINT('',(-725.,-505.,-297.));
#5839=CARTESIAN_POINT('',(-725.,-505.,-297.));
#5840=CARTESIAN_POINT('',(-355.,-505.,-297.));
#5841=CARTESIAN_POINT('',(-355.,-505.,-297.));
#5842=CARTESIAN_POINT('',(-355.,-535.,-297.));
#5843=CARTESIAN_POINT('Origin',(247.,-535.,300.));
#5844=CARTESIAN_POINT('',(247.,-505.,-250.));
#5845=CARTESIAN_POINT('',(247.,-535.,-250.));
#5846=CARTESIAN_POINT('',(247.,-505.,250.));
#5847=CARTESIAN_POINT('',(247.,-505.,-250.));
#5848=CARTESIAN_POINT('',(247.,-505.,250.));
#5849=CARTESIAN_POINT('',(247.,-288.,297.));
#5850=CARTESIAN_POINT('Origin',(0.,-288.,0.));
#5851=CARTESIAN_POINT('',(-500.,-288.,35.));
#5852=CARTESIAN_POINT('Origin',(-500.,-288.,-6.12323399573677E-14));
#5853=CARTESIAN_POINT('',(-4.28626379701574E-15,-288.,35.));
#5854=CARTESIAN_POINT('Origin',(0.,-288.,0.));
#5855=CARTESIAN_POINT('Origin',(-355.,-535.,-300.));
#5856=CARTESIAN_POINT('',(-355.,-537.,300.));
#5857=CARTESIAN_POINT('',(-355.,-535.,300.));
#5858=CARTESIAN_POINT('',(-355.,-537.,327.60400694353));
#5859=CARTESIAN_POINT('',(-355.,-537.,327.60400694353));
#5860=CARTESIAN_POINT('',(-355.,-534.,327.60400694353));
#5861=CARTESIAN_POINT('',(-355.,-534.,327.60400694353));
#5862=CARTESIAN_POINT('',(-355.,-534.,327.60400694353));
#5863=CARTESIAN_POINT('',(-355.,-505.,297.));
#5864=CARTESIAN_POINT('Origin',(-355.,-505.,-300.));
#5865=CARTESIAN_POINT('',(-725.,-505.,299.));
#5866=CARTESIAN_POINT('Origin',(-726.,-505.,299.));
#5867=CARTESIAN_POINT('',(-725.,-505.,297.));
#5868=CARTESIAN_POINT('Origin',(-725.,-505.,-300.));
#5869=CARTESIAN_POINT('',(-725.,-533.,299.));
#5870=CARTESIAN_POINT('',(-725.,-505.,299.));
#5871=CARTESIAN_POINT('',(-725.,-535.,301.));
#5872=CARTESIAN_POINT('Origin',(-725.,-533.,301.));
#5873=CARTESIAN_POINT('',(-725.,-535.,327.60400694353));
#5874=CARTESIAN_POINT('',(-725.,-535.,301.));
#5875=CARTESIAN_POINT('',(-725.,-537.,327.60400694353));
#5876=CARTESIAN_POINT('',(-725.,-535.,327.60400694353));
#5877=CARTESIAN_POINT('',(-725.,-537.,300.));
#5878=CARTESIAN_POINT('',(-725.,-537.,300.));
#5879=CARTESIAN_POINT('',(-725.,-535.,300.));
#5880=CARTESIAN_POINT('Origin',(175.,-505.,-300.));
#5881=CARTESIAN_POINT('',(175.,-533.,299.));
#5882=CARTESIAN_POINT('',(175.,-535.,301.));
#5883=CARTESIAN_POINT('Origin',(175.,-533.,301.));
#5884=CARTESIAN_POINT('',(175.,-505.,299.));
#5885=CARTESIAN_POINT('',(175.,-533.,299.));
#5886=CARTESIAN_POINT('',(175.,-505.,297.));
#5887=CARTESIAN_POINT('',(175.,-537.,300.));
#5888=CARTESIAN_POINT('',(175.,-535.,300.));
#5889=CARTESIAN_POINT('',(175.,-537.,327.60400694353));
#5890=CARTESIAN_POINT('',(175.,-537.,327.60400694353));
#5891=CARTESIAN_POINT('',(175.,-535.,327.60400694353));
#5892=CARTESIAN_POINT('',(175.,-535.,327.60400694353));
#5893=CARTESIAN_POINT('',(175.,-535.,327.60400694353));
#5894=CARTESIAN_POINT('Origin',(-195.,-505.,-300.));
#5895=CARTESIAN_POINT('',(-195.,-505.,297.));
#5896=CARTESIAN_POINT('Origin',(176.,-505.,299.));
#5897=CARTESIAN_POINT('Origin',(-195.,-535.,-300.));
#5898=CARTESIAN_POINT('',(-195.,-534.,327.60400694353));
#5899=CARTESIAN_POINT('',(-195.,-534.,300.));
#5900=CARTESIAN_POINT('',(-195.,-537.,327.60400694353));
#5901=CARTESIAN_POINT('',(-195.,-534.,327.60400694353));
#5902=CARTESIAN_POINT('',(-195.,-537.,300.));
#5903=CARTESIAN_POINT('',(-195.,-537.,300.));
#5904=CARTESIAN_POINT('',(-195.,-535.,300.));
#5905=CARTESIAN_POINT('Origin',(-355.,-535.,-300.));
#5906=CARTESIAN_POINT('',(-355.,-505.,-300.));
#5907=CARTESIAN_POINT('',(-355.,-534.,-327.60400694353));
#5908=CARTESIAN_POINT('',(-355.,-534.,-300.));
#5909=CARTESIAN_POINT('',(-355.,-537.,-327.60400694353));
#5910=CARTESIAN_POINT('',(-355.,-534.,-327.60400694353));
#5911=CARTESIAN_POINT('',(-355.,-537.,-300.));
#5912=CARTESIAN_POINT('',(-355.,-537.,-300.));
#5913=CARTESIAN_POINT('',(-355.,-535.,-300.));
#5914=CARTESIAN_POINT('Origin',(-355.,-505.,-300.));
#5915=CARTESIAN_POINT('',(-725.,-505.,-299.));
#5916=CARTESIAN_POINT('',(-725.,-505.,-299.));
#5917=CARTESIAN_POINT('Origin',(-726.,-505.,-299.));
#5918=CARTESIAN_POINT('Origin',(-725.,-505.,-300.));
#5919=CARTESIAN_POINT('',(-725.,-533.,-299.));
#5920=CARTESIAN_POINT('',(-725.,-535.,-301.));
#5921=CARTESIAN_POINT('Origin',(-725.,-533.,-301.));
#5922=CARTESIAN_POINT('',(-725.,-505.,-299.));
#5923=CARTESIAN_POINT('',(-725.,-537.,-300.));
#5924=CARTESIAN_POINT('',(-725.,-535.,-300.));
#5925=CARTESIAN_POINT('',(-725.,-537.,-327.60400694353));
#5926=CARTESIAN_POINT('',(-725.,-537.,-327.60400694353));
#5927=CARTESIAN_POINT('',(-725.,-535.,-327.60400694353));
#5928=CARTESIAN_POINT('',(-725.,-535.,-327.60400694353));
#5929=CARTESIAN_POINT('',(-725.,-535.,-327.60400694353));
#5930=CARTESIAN_POINT('Origin',(-195.,-535.,-300.));
#5931=CARTESIAN_POINT('',(-195.,-537.,-300.));
#5932=CARTESIAN_POINT('',(-195.,-535.,-300.));
#5933=CARTESIAN_POINT('',(-195.,-537.,-327.60400694353));
#5934=CARTESIAN_POINT('',(-195.,-537.,-327.60400694353));
#5935=CARTESIAN_POINT('',(-195.,-534.,-327.60400694353));
#5936=CARTESIAN_POINT('',(-195.,-534.,-327.60400694353));
#5937=CARTESIAN_POINT('',(-195.,-534.,-327.60400694353));
#5938=CARTESIAN_POINT('',(-195.,-505.,-300.));
#5939=CARTESIAN_POINT('Origin',(175.,-505.,-300.));
#5940=CARTESIAN_POINT('',(175.,-505.,-299.));
#5941=CARTESIAN_POINT('',(175.,-505.,-299.));
#5942=CARTESIAN_POINT('',(175.,-533.,-299.));
#5943=CARTESIAN_POINT('',(175.,-533.,-299.));
#5944=CARTESIAN_POINT('',(175.,-535.,-301.));
#5945=CARTESIAN_POINT('Origin',(175.,-533.,-301.));
#5946=CARTESIAN_POINT('',(175.,-535.,-327.60400694353));
#5947=CARTESIAN_POINT('',(175.,-535.,-301.));
#5948=CARTESIAN_POINT('',(175.,-537.,-327.60400694353));
#5949=CARTESIAN_POINT('',(175.,-535.,-327.60400694353));
#5950=CARTESIAN_POINT('',(175.,-537.,-300.));
#5951=CARTESIAN_POINT('',(175.,-537.,-300.));
#5952=CARTESIAN_POINT('',(175.,-535.,-300.));
#5953=CARTESIAN_POINT('Origin',(-195.,-505.,-300.));
#5954=CARTESIAN_POINT('Origin',(176.,-505.,-299.));
#5955=CARTESIAN_POINT('Origin',(0.,-330.693069306929,100.));
#5956=CARTESIAN_POINT('',(205.,-330.693069306929,297.));
#5957=CARTESIAN_POINT('',(-115.,-330.693069306929,297.));
#5958=CARTESIAN_POINT('Origin',(205.,-3.67089871045415E-14,100.));
#5959=CARTESIAN_POINT('',(205.,-485.693069306929,297.));
#5960=CARTESIAN_POINT('Origin',(0.,-485.693069306929,100.));
#5961=CARTESIAN_POINT('',(-115.,-485.693069306929,297.));
#5962=CARTESIAN_POINT('Origin',(-115.,-1.02964232122494E-14,100.));
#5963=CARTESIAN_POINT('Origin',(-435.,0.,100.));
#5964=CARTESIAN_POINT('',(-435.,-485.693069306929,297.));
#5965=CARTESIAN_POINT('',(-435.,-330.693069306929,297.));
#5966=CARTESIAN_POINT('Origin',(0.,-485.693069306929,100.));
#5967=CARTESIAN_POINT('',(-755.,-485.693069306929,297.));
#5968=CARTESIAN_POINT('Origin',(-755.,0.,100.));
#5969=CARTESIAN_POINT('',(-755.,-330.693069306929,297.));
#5970=CARTESIAN_POINT('Origin',(0.,-330.693069306929,100.));
#5971=CARTESIAN_POINT('Origin',(-120.,-490.693069306929,280.));
#5972=CARTESIAN_POINT('',(-122.,-490.693069306929,280.));
#5973=CARTESIAN_POINT('Origin',(210.,-490.693069306929,280.));
#5974=CARTESIAN_POINT('',(208.,-490.693069306929,280.));
#5975=CARTESIAN_POINT('Origin',(-120.,-325.693069306929,280.));
#5976=CARTESIAN_POINT('',(-122.,-325.693069306929,280.));
#5977=CARTESIAN_POINT('Origin',(210.,-325.693069306929,280.));
#5978=CARTESIAN_POINT('',(208.,-325.693069306929,280.));
#5979=CARTESIAN_POINT('Origin',(250.,-505.,250.));
#5980=CARTESIAN_POINT('',(249.,-505.,250.));
#5981=CARTESIAN_POINT('',(249.,-505.,250.));
#5982=CARTESIAN_POINT('',(249.,-533.,250.));
#5983=CARTESIAN_POINT('',(249.,-533.,250.));
#5984=CARTESIAN_POINT('',(251.,-535.,250.));
#5985=CARTESIAN_POINT('Origin',(251.,-533.,250.));
#5986=CARTESIAN_POINT('',(277.60400694353,-535.,250.));
#5987=CARTESIAN_POINT('',(251.,-535.,250.));
#5988=CARTESIAN_POINT('',(277.60400694353,-537.,250.));
#5989=CARTESIAN_POINT('',(277.60400694353,-535.,250.));
#5990=CARTESIAN_POINT('',(250.,-537.,250.));
#5991=CARTESIAN_POINT('',(250.,-537.,250.));
#5992=CARTESIAN_POINT('',(250.,-535.,250.));
#5993=CARTESIAN_POINT('Origin',(250.,-505.,-250.));
#5994=CARTESIAN_POINT('',(249.,-505.,-250.));
#5995=CARTESIAN_POINT('',(249.,-505.,-250.));
#5996=CARTESIAN_POINT('Origin',(249.,-505.,-251.));
#5997=CARTESIAN_POINT('Origin',(249.,-505.,251.));
#5998=CARTESIAN_POINT('Origin',(250.,-505.,-250.));
#5999=CARTESIAN_POINT('',(249.,-533.,-250.));
#6000=CARTESIAN_POINT('',(251.,-535.,-250.));
#6001=CARTESIAN_POINT('Origin',(251.,-533.,-250.));
#6002=CARTESIAN_POINT('',(249.,-505.,-250.));
#6003=CARTESIAN_POINT('',(250.,-537.,-250.));
#6004=CARTESIAN_POINT('',(250.,-535.,-250.));
#6005=CARTESIAN_POINT('',(277.60400694353,-537.,-250.));
#6006=CARTESIAN_POINT('',(277.60400694353,-537.,-250.));
#6007=CARTESIAN_POINT('',(277.60400694353,-535.,-250.));
#6008=CARTESIAN_POINT('',(277.60400694353,-535.,-250.));
#6009=CARTESIAN_POINT('',(277.60400694353,-535.,-250.));
#6010=CARTESIAN_POINT('Origin',(250.,-505.,-250.));
#6011=CARTESIAN_POINT('',(-799.,-505.,-250.));
#6012=CARTESIAN_POINT('',(-797.,-505.,-250.));
#6013=CARTESIAN_POINT('',(-799.,-533.,-250.));
#6014=CARTESIAN_POINT('',(-799.,-533.,-250.));
#6015=CARTESIAN_POINT('',(-801.,-535.,-250.));
#6016=CARTESIAN_POINT('Origin',(-801.,-533.,-250.));
#6017=CARTESIAN_POINT('',(-827.604006943529,-535.,-250.));
#6018=CARTESIAN_POINT('',(-801.,-535.,-250.));
#6019=CARTESIAN_POINT('',(-827.604006943529,-537.,-250.));
#6020=CARTESIAN_POINT('',(-827.604006943529,-535.,-250.));
#6021=CARTESIAN_POINT('',(-800.,-537.,-250.));
#6022=CARTESIAN_POINT('',(-800.,-537.,-250.));
#6023=CARTESIAN_POINT('',(-800.,-535.,-250.));
#6024=CARTESIAN_POINT('Origin',(250.,-505.,-250.));
#6025=CARTESIAN_POINT('',(-799.,-505.,250.));
#6026=CARTESIAN_POINT('',(-797.,-505.,250.));
#6027=CARTESIAN_POINT('Origin',(-799.,-505.,251.));
#6028=CARTESIAN_POINT('Origin',(-799.,-505.,-251.));
#6029=CARTESIAN_POINT('Origin',(250.,-505.,250.));
#6030=CARTESIAN_POINT('',(-799.,-533.,250.));
#6031=CARTESIAN_POINT('',(-801.,-535.,250.));
#6032=CARTESIAN_POINT('Origin',(-801.,-533.,250.));
#6033=CARTESIAN_POINT('',(-799.,-505.,250.));
#6034=CARTESIAN_POINT('',(-800.,-537.,250.));
#6035=CARTESIAN_POINT('',(-800.,-535.,250.));
#6036=CARTESIAN_POINT('',(-827.604006943529,-537.,250.));
#6037=CARTESIAN_POINT('',(-827.604006943529,-537.,250.));
#6038=CARTESIAN_POINT('',(-827.604006943529,-535.,250.));
#6039=CARTESIAN_POINT('',(-827.604006943529,-535.,250.));
#6040=CARTESIAN_POINT('',(-827.604006943529,-535.,250.));
#6041=CARTESIAN_POINT('Origin',(-725.,-534.,327.60400694353));
#6042=CARTESIAN_POINT('',(-827.604006943529,-535.,327.60400694353));
#6043=CARTESIAN_POINT('',(-725.,-535.,327.60400694353));
#6044=CARTESIAN_POINT('',(-827.604006943529,-537.,327.60400694353));
#6045=CARTESIAN_POINT('',(-827.604006943529,-535.,327.60400694353));
#6046=CARTESIAN_POINT('',(-725.,-537.,327.60400694353));
#6047=CARTESIAN_POINT('Origin',(-800.,-534.,300.));
#6048=CARTESIAN_POINT('',(-800.,-537.,300.));
#6049=CARTESIAN_POINT('',(-800.,-535.,300.));
#6050=CARTESIAN_POINT('',(-800.,-537.,300.));
#6051=CARTESIAN_POINT('Origin',(-800.,-534.,300.));
#6052=CARTESIAN_POINT('',(-800.,-537.,250.));
#6053=CARTESIAN_POINT('Origin',(-827.604006943529,-534.,327.60400694353));
#6054=CARTESIAN_POINT('',(-827.604006943529,-535.,327.60400694353));
#6055=CARTESIAN_POINT('',(-827.604006943529,-537.,327.60400694353));
#6056=CARTESIAN_POINT('Origin',(0.,-534.,0.));
#6057=CARTESIAN_POINT('',(-801.,-534.,251.));
#6058=CARTESIAN_POINT('',(-826.60400694353,-534.,251.));
#6059=CARTESIAN_POINT('',(-826.60400694353,-534.,251.));
#6060=CARTESIAN_POINT('',(-826.60400694353,-534.,326.60400694353));
#6061=CARTESIAN_POINT('',(-826.60400694353,-534.,326.60400694353));
#6062=CARTESIAN_POINT('',(-726.,-534.,326.60400694353));
#6063=CARTESIAN_POINT('',(-726.,-534.,326.60400694353));
#6064=CARTESIAN_POINT('',(-726.,-534.,301.));
#6065=CARTESIAN_POINT('',(-726.,-534.,301.));
#6066=CARTESIAN_POINT('',(-801.,-534.,301.));
#6067=CARTESIAN_POINT('',(-801.,-534.,301.));
#6068=CARTESIAN_POINT('',(-801.,-534.,251.));
#6069=CARTESIAN_POINT('Origin',(0.,-537.,0.));
#6070=CARTESIAN_POINT('Origin',(-800.,-534.,-300.));
#6071=CARTESIAN_POINT('',(-800.,-537.,-300.));
#6072=CARTESIAN_POINT('',(-800.,-535.,-300.));
#6073=CARTESIAN_POINT('',(-725.,-537.,-300.));
#6074=CARTESIAN_POINT('Origin',(-725.,-534.,-327.60400694353));
#6075=CARTESIAN_POINT('',(-827.604006943529,-535.,-327.60400694353));
#6076=CARTESIAN_POINT('',(-827.604006943529,-537.,-327.60400694353));
#6077=CARTESIAN_POINT('',(-827.604006943529,-535.,-327.60400694353));
#6078=CARTESIAN_POINT('',(-827.604006943529,-535.,-327.60400694353));
#6079=CARTESIAN_POINT('',(-827.604006943529,-537.,-327.60400694353));
#6080=CARTESIAN_POINT('Origin',(-827.604006943529,-534.,-327.60400694353));
#6081=CARTESIAN_POINT('',(-827.604006943529,-535.,-250.));
#6082=CARTESIAN_POINT('',(-827.604006943529,-537.,-250.));
#6083=CARTESIAN_POINT('Origin',(-800.,-534.,-300.));
#6084=CARTESIAN_POINT('',(-800.,-537.,-300.));
#6085=CARTESIAN_POINT('Origin',(0.,-534.,0.));
#6086=CARTESIAN_POINT('',(-826.60400694353,-534.,-251.));
#6087=CARTESIAN_POINT('',(-801.,-534.,-251.));
#6088=CARTESIAN_POINT('',(-801.,-534.,-251.));
#6089=CARTESIAN_POINT('',(-801.,-534.,-301.));
#6090=CARTESIAN_POINT('',(-801.,-534.,-301.));
#6091=CARTESIAN_POINT('',(-726.,-534.,-301.));
#6092=CARTESIAN_POINT('',(-726.,-534.,-301.));
#6093=CARTESIAN_POINT('',(-726.,-534.,-326.60400694353));
#6094=CARTESIAN_POINT('',(-726.,-534.,-326.60400694353));
#6095=CARTESIAN_POINT('',(-826.60400694353,-534.,-326.60400694353));
#6096=CARTESIAN_POINT('',(-826.60400694353,-534.,-326.60400694353));
#6097=CARTESIAN_POINT('',(-826.60400694353,-534.,-251.));
#6098=CARTESIAN_POINT('Origin',(0.,-537.,0.));
#6099=CARTESIAN_POINT('Origin',(250.,-534.,-300.));
#6100=CARTESIAN_POINT('',(250.,-537.,-300.));
#6101=CARTESIAN_POINT('',(250.,-535.,-300.));
#6102=CARTESIAN_POINT('',(250.,-537.,-250.));
#6103=CARTESIAN_POINT('Origin',(277.60400694353,-534.,-327.60400694353));
#6104=CARTESIAN_POINT('',(277.60400694353,-535.,-327.60400694353));
#6105=CARTESIAN_POINT('',(277.60400694353,-537.,-327.60400694353));
#6106=CARTESIAN_POINT('',(277.60400694353,-535.,-327.60400694353));
#6107=CARTESIAN_POINT('',(277.60400694353,-535.,-327.60400694353));
#6108=CARTESIAN_POINT('',(277.60400694353,-537.,-327.60400694353));
#6109=CARTESIAN_POINT('Origin',(175.,-534.,-327.60400694353));
#6110=CARTESIAN_POINT('',(175.,-535.,-327.60400694353));
#6111=CARTESIAN_POINT('',(175.,-537.,-327.60400694353));
#6112=CARTESIAN_POINT('Origin',(250.,-534.,-300.));
#6113=CARTESIAN_POINT('',(250.,-537.,-300.));
#6114=CARTESIAN_POINT('Origin',(0.,-534.,0.));
#6115=CARTESIAN_POINT('',(176.,-534.,-326.60400694353));
#6116=CARTESIAN_POINT('',(176.,-534.,-301.));
#6117=CARTESIAN_POINT('',(176.,-534.,-301.));
#6118=CARTESIAN_POINT('',(251.,-534.,-301.));
#6119=CARTESIAN_POINT('',(251.,-534.,-301.));
#6120=CARTESIAN_POINT('',(251.,-534.,-251.));
#6121=CARTESIAN_POINT('',(251.,-534.,-251.));
#6122=CARTESIAN_POINT('',(276.60400694353,-534.,-251.));
#6123=CARTESIAN_POINT('',(276.60400694353,-534.,-251.));
#6124=CARTESIAN_POINT('',(276.60400694353,-534.,-326.60400694353));
#6125=CARTESIAN_POINT('',(276.60400694353,-534.,-326.60400694353));
#6126=CARTESIAN_POINT('',(176.,-534.,-326.60400694353));
#6127=CARTESIAN_POINT('Origin',(0.,-537.,0.));
#6128=CARTESIAN_POINT('Origin',(250.,-534.,300.));
#6129=CARTESIAN_POINT('',(250.,-537.,300.));
#6130=CARTESIAN_POINT('',(250.,-535.,300.));
#6131=CARTESIAN_POINT('',(175.,-537.,300.));
#6132=CARTESIAN_POINT('Origin',(175.,-534.,327.60400694353));
#6133=CARTESIAN_POINT('',(277.60400694353,-535.,327.60400694353));
#6134=CARTESIAN_POINT('',(277.60400694353,-537.,327.60400694353));
#6135=CARTESIAN_POINT('',(277.60400694353,-535.,327.60400694353));
#6136=CARTESIAN_POINT('',(277.60400694353,-535.,327.60400694353));
#6137=CARTESIAN_POINT('',(277.60400694353,-537.,327.60400694353));
#6138=CARTESIAN_POINT('Origin',(277.60400694353,-534.,327.60400694353));
#6139=CARTESIAN_POINT('',(277.60400694353,-535.,250.));
#6140=CARTESIAN_POINT('',(277.60400694353,-537.,250.));
#6141=CARTESIAN_POINT('Origin',(250.,-534.,300.));
#6142=CARTESIAN_POINT('',(250.,-537.,300.));
#6143=CARTESIAN_POINT('Origin',(0.,-534.,0.));
#6144=CARTESIAN_POINT('',(276.60400694353,-534.,251.));
#6145=CARTESIAN_POINT('',(251.,-534.,251.));
#6146=CARTESIAN_POINT('',(251.,-534.,251.));
#6147=CARTESIAN_POINT('',(251.,-534.,301.));
#6148=CARTESIAN_POINT('',(251.,-534.,301.));
#6149=CARTESIAN_POINT('',(176.,-534.,301.));
#6150=CARTESIAN_POINT('',(176.,-534.,301.));
#6151=CARTESIAN_POINT('',(176.,-534.,326.60400694353));
#6152=CARTESIAN_POINT('',(176.,-534.,326.60400694353));
#6153=CARTESIAN_POINT('',(276.60400694353,-534.,326.60400694353));
#6154=CARTESIAN_POINT('',(276.60400694353,-534.,326.60400694353));
#6155=CARTESIAN_POINT('',(276.60400694353,-534.,251.));
#6156=CARTESIAN_POINT('Origin',(0.,-537.,0.));
#6157=CARTESIAN_POINT('Origin',(-355.,-534.,-300.));
#6158=CARTESIAN_POINT('',(-195.,-537.,-300.));
#6159=CARTESIAN_POINT('Origin',(-355.,-534.,-327.60400694353));
#6160=CARTESIAN_POINT('',(-355.,-537.,-327.60400694353));
#6161=CARTESIAN_POINT('',(-355.,-534.,-327.60400694353));
#6162=CARTESIAN_POINT('Origin',(0.,-534.,0.));
#6163=CARTESIAN_POINT('Origin',(0.,-537.,0.));
#6164=CARTESIAN_POINT('Origin',(-355.,-534.,327.60400694353));
#6165=CARTESIAN_POINT('',(-195.,-537.,327.60400694353));
#6166=CARTESIAN_POINT('',(-195.,-534.,327.60400694353));
#6167=CARTESIAN_POINT('Origin',(-355.,-534.,300.));
#6168=CARTESIAN_POINT('',(-355.,-537.,300.));
#6169=CARTESIAN_POINT('Origin',(0.,-534.,0.));
#6170=CARTESIAN_POINT('Origin',(0.,-537.,0.));
#6171=CARTESIAN_POINT('Origin',(-726.,-535.,-300.));
#6172=CARTESIAN_POINT('Origin',(-726.,-535.,-301.));
#6173=CARTESIAN_POINT('Origin',(-726.,-535.,-326.60400694353));
#6174=CARTESIAN_POINT('Origin',(-726.,-535.,-299.));
#6175=CARTESIAN_POINT('Origin',(-726.,-533.,-299.));
#6176=CARTESIAN_POINT('Origin',(-725.,-535.,-326.60400694353));
#6177=CARTESIAN_POINT('Origin',(-826.60400694353,-535.,-326.60400694353));
#6178=CARTESIAN_POINT('Origin',(-726.,-533.,-301.));
#6179=CARTESIAN_POINT('Origin',(-726.,-533.,-301.));
#6180=CARTESIAN_POINT('Origin',(-826.60400694353,-535.,-327.60400694353));
#6181=CARTESIAN_POINT('Origin',(-826.604006943529,-535.,-251.));
#6182=CARTESIAN_POINT('Origin',(-800.,-533.,-301.));
#6183=CARTESIAN_POINT('Origin',(-801.,-533.,-301.));
#6184=CARTESIAN_POINT('Origin',(250.,-535.,-251.));
#6185=CARTESIAN_POINT('Origin',(-801.,-535.,-251.));
#6186=CARTESIAN_POINT('Origin',(-801.,-533.,300.));
#6187=CARTESIAN_POINT('Origin',(-801.,-533.,-251.));
#6188=CARTESIAN_POINT('Origin',(-801.,-533.,-251.));
#6189=CARTESIAN_POINT('Origin',(-799.,-533.,-251.));
#6190=CARTESIAN_POINT('Origin',(-799.,-535.,-251.));
#6191=CARTESIAN_POINT('Origin',(250.,-535.,-251.));
#6192=CARTESIAN_POINT('Origin',(251.,-535.,-251.));
#6193=CARTESIAN_POINT('Origin',(276.60400694353,-535.,-251.));
#6194=CARTESIAN_POINT('Origin',(249.,-535.,-251.));
#6195=CARTESIAN_POINT('Origin',(249.,-533.,-251.));
#6196=CARTESIAN_POINT('Origin',(276.60400694353,-535.,-327.60400694353));
#6197=CARTESIAN_POINT('Origin',(276.60400694353,-535.,-326.60400694353));
#6198=CARTESIAN_POINT('Origin',(251.,-533.,-251.));
#6199=CARTESIAN_POINT('Origin',(251.,-533.,-251.));
#6200=CARTESIAN_POINT('Origin',(175.,-535.,-326.60400694353));
#6201=CARTESIAN_POINT('Origin',(176.,-535.,-326.60400694353));
#6202=CARTESIAN_POINT('Origin',(251.,-533.,300.));
#6203=CARTESIAN_POINT('Origin',(251.,-533.,-301.));
#6204=CARTESIAN_POINT('Origin',(176.,-535.,-300.));
#6205=CARTESIAN_POINT('Origin',(176.,-535.,-301.));
#6206=CARTESIAN_POINT('Origin',(-800.,-533.,-301.));
#6207=CARTESIAN_POINT('Origin',(176.,-533.,-301.));
#6208=CARTESIAN_POINT('Origin',(176.,-533.,-301.));
#6209=CARTESIAN_POINT('Origin',(176.,-533.,-299.));
#6210=CARTESIAN_POINT('Origin',(176.,-535.,-299.));
#6211=CARTESIAN_POINT('Origin',(176.,-535.,-300.));
#6212=CARTESIAN_POINT('Origin',(176.,-535.,301.));
#6213=CARTESIAN_POINT('Origin',(176.,-535.,326.60400694353));
#6214=CARTESIAN_POINT('Origin',(176.,-505.,299.));
#6215=CARTESIAN_POINT('Origin',(176.,-533.,299.));
#6216=CARTESIAN_POINT('Origin',(175.,-535.,326.60400694353));
#6217=CARTESIAN_POINT('Origin',(276.60400694353,-535.,326.60400694353));
#6218=CARTESIAN_POINT('Origin',(176.,-533.,301.));
#6219=CARTESIAN_POINT('Origin',(176.,-533.,301.));
#6220=CARTESIAN_POINT('Origin',(276.60400694353,-535.,327.60400694353));
#6221=CARTESIAN_POINT('Origin',(276.60400694353,-535.,251.));
#6222=CARTESIAN_POINT('Origin',(-800.,-533.,301.));
#6223=CARTESIAN_POINT('Origin',(251.,-533.,301.));
#6224=CARTESIAN_POINT('Origin',(250.,-535.,251.));
#6225=CARTESIAN_POINT('Origin',(251.,-535.,251.));
#6226=CARTESIAN_POINT('Origin',(251.,-533.,300.));
#6227=CARTESIAN_POINT('Origin',(251.,-533.,251.));
#6228=CARTESIAN_POINT('Origin',(251.,-533.,251.));
#6229=CARTESIAN_POINT('Origin',(249.,-533.,251.));
#6230=CARTESIAN_POINT('Origin',(249.,-535.,251.));
#6231=CARTESIAN_POINT('Origin',(-726.,-505.,299.));
#6232=CARTESIAN_POINT('Origin',(-726.,-533.,299.));
#6233=CARTESIAN_POINT('Origin',(-726.,-535.,-300.));
#6234=CARTESIAN_POINT('Origin',(-726.,-535.,326.60400694353));
#6235=CARTESIAN_POINT('Origin',(-726.,-535.,301.));
#6236=CARTESIAN_POINT('Origin',(-726.,-533.,301.));
#6237=CARTESIAN_POINT('Origin',(-726.,-533.,301.));
#6238=CARTESIAN_POINT('Origin',(-725.,-535.,326.60400694353));
#6239=CARTESIAN_POINT('Origin',(-826.60400694353,-535.,326.60400694353));
#6240=CARTESIAN_POINT('Origin',(-800.,-533.,301.));
#6241=CARTESIAN_POINT('Origin',(-801.,-533.,301.));
#6242=CARTESIAN_POINT('Origin',(-826.60400694353,-535.,327.60400694353));
#6243=CARTESIAN_POINT('Origin',(-826.604006943529,-535.,251.));
#6244=CARTESIAN_POINT('Origin',(-801.,-533.,300.));
#6245=CARTESIAN_POINT('Origin',(-801.,-533.,251.));
#6246=CARTESIAN_POINT('Origin',(250.,-535.,251.));
#6247=CARTESIAN_POINT('Origin',(-801.,-535.,251.));
#6248=CARTESIAN_POINT('Origin',(-801.,-533.,251.));
#6249=CARTESIAN_POINT('Origin',(-799.,-533.,251.));
#6250=CARTESIAN_POINT('Origin',(-799.,-535.,251.));
#6251=CARTESIAN_POINT('Origin',(0.,175.,0.));
#6252=CARTESIAN_POINT('',(-4.28626379701574E-15,175.,35.));
#6253=CARTESIAN_POINT('Origin',(-500.,175.,-6.12323399573677E-14));
#6254=CARTESIAN_POINT('',(-500.,175.,35.));
#6774=UNCERTAINTY_MEASURE_WITH_UNIT(LENGTH_MEASURE(0.01),#6790,
'DISTANCE_ACCURACY_VALUE',
'Maximum model space distance between geometric entities at asserted c
onnectivities');
#6780=UNCERTAINTY_MEASURE_WITH_UNIT(LENGTH_MEASURE(0.01),#6790,
'DISTANCE_ACCURACY_VALUE',
'Maximum model space distance between geometric entities at asserted c
onnectivities');
#6783=(
GEOMETRIC_REPRESENTATION_CONTEXT(3)
GLOBAL_UNCERTAINTY_ASSIGNED_CONTEXT((#6774))
GLOBAL_UNIT_ASSIGNED_CONTEXT((#6790,#6792,#6793))
REPRESENTATION_CONTEXT('','3D')
);
#6789=(
GEOMETRIC_REPRESENTATION_CONTEXT(3)
GLOBAL_UNCERTAINTY_ASSIGNED_CONTEXT((#6780))
GLOBAL_UNIT_ASSIGNED_CONTEXT((#6790,#6792,#6793))
REPRESENTATION_CONTEXT('','3D')
);
#6790=(
LENGTH_UNIT()
NAMED_UNIT(*)
SI_UNIT(.MILLI.,.METRE.)
);
#6792=(
NAMED_UNIT(*)
PLANE_ANGLE_UNIT()
SI_UNIT($,.RADIAN.)
);
#6793=(
NAMED_UNIT(*)
SI_UNIT($,.STERADIAN.)
SOLID_ANGLE_UNIT()
);
#6796=SHAPE_DEFINITION_REPRESENTATION(#6804,#6821);
#6804=PRODUCT_DEFINITION_SHAPE('',$,#6830);
#6821=SHAPE_REPRESENTATION('',(#4036),#6783);
#6827=PRODUCT_DEFINITION_CONTEXT('part definition',#6853,'design');
#6830=PRODUCT_DEFINITION('Bottom Base','Bottom Base',#6838,#6827);
#6838=PRODUCT_DEFINITION_FORMATION('',$,#6857);
#6853=APPLICATION_CONTEXT(
'Core Data for Automotive Mechanical Design Process');
#6854=PRODUCT_CONTEXT('part definition',#6853,'mechanical');
#6857=PRODUCT('Bottom Base','Bottom Base',$,(#6854));
#6863=PRESENTATION_STYLE_ASSIGNMENT((#6865));
#6865=SURFACE_STYLE_USAGE(.BOTH.,#6867);
#6867=SURFACE_SIDE_STYLE('',(#6869));
#6869=SURFACE_STYLE_FILL_AREA(#6871);
#6871=FILL_AREA_STYLE('Steel - Satin',(#6873));
#6873=FILL_AREA_STYLE_COLOUR('Steel - Satin',#6875);
#6875=COLOUR_RGB('Steel - Satin',0.627450980392157,0.627450980392157,0.627450980392157);
ENDSEC;
END-ISO-10303-21;
